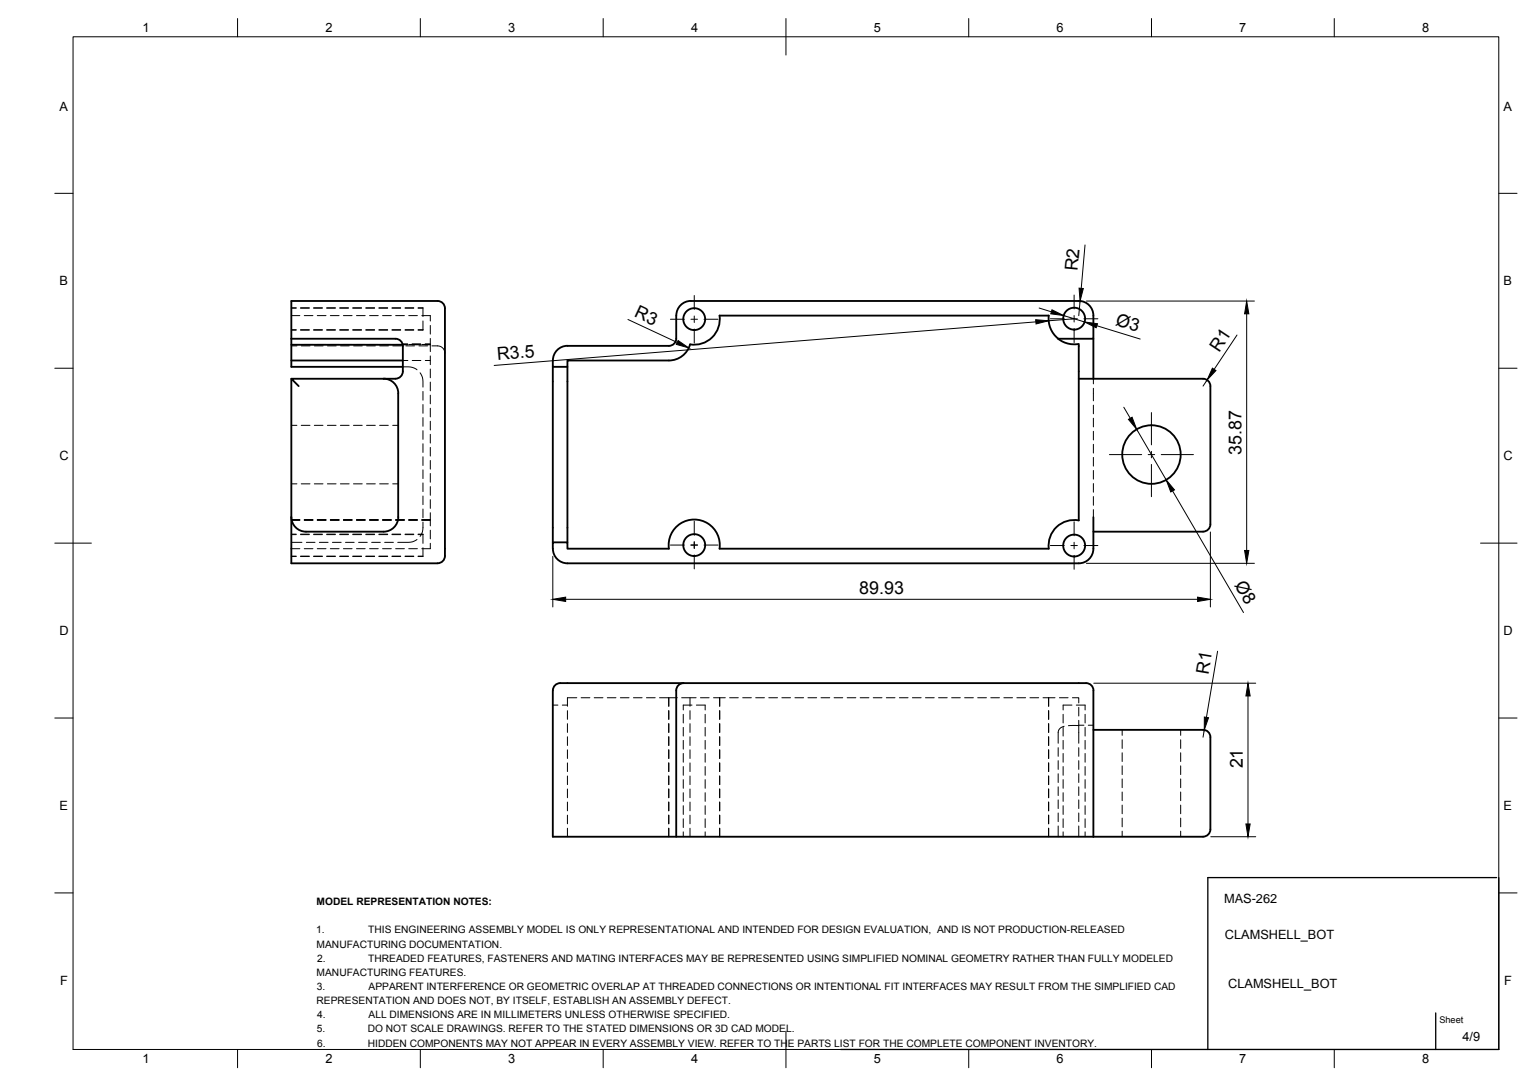
ISO-10303-21;
HEADER;
/* Generated by software containing ST-Developer
 * from STEP Tools, Inc. (www.steptools.com) 
 */

FILE_DESCRIPTION(
/* description */ (''),
/* implementation_level */ '2;1');

FILE_NAME(
/* name */ 'CLAMSHELL_BOT.step',
/* time_stamp */ '2026-10-07T02:13:48+06:00',
/* author */ (''),
/* organization */ (''),
/* preprocessor_version */ 'ST-DEVELOPER v20.2',
/* originating_system */ 'Autodesk Translation Framework v15.15.0.0',
/* authorisation */ '');

FILE_SCHEMA (('AUTOMOTIVE_DESIGN { 1 0 10303 214 3 1 1 }'));
ENDSEC;

DATA;
#10=MECHANICAL_DESIGN_GEOMETRIC_PRESENTATION_REPRESENTATION('',(#115),#17042);
#91=SHAPE_REPRESENTATION_RELATIONSHIP('SRR','None',#17087,#103);
#103=ADVANCED_BREP_SHAPE_REPRESENTATION('',(#127),#17031);
#115=STYLED_ITEM('',(#17154),#127);
#127=MANIFOLD_SOLID_BREP('Body1',#8116);
#142=FACE_BOUND('',#1059,.T.);
#143=FACE_BOUND('',#1060,.T.);
#144=FACE_BOUND('',#1071,.T.);
#145=FACE_BOUND('',#1079,.T.);
#146=FACE_BOUND('',#1085,.T.);
#147=FACE_BOUND('',#1086,.T.);
#180=(
BOUNDED_SURFACE()
B_SPLINE_SURFACE(2,2,((#12432,#12433,#12434),(#12435,#12436,#12437),(#12438,
#12439,#12440)),.UNSPECIFIED.,.F.,.F.,.F.)
B_SPLINE_SURFACE_WITH_KNOTS((3,3),(3,3),(0.,1.5707963267949),(-1.5707963267949,
0.),.UNSPECIFIED.)
GEOMETRIC_REPRESENTATION_ITEM()
RATIONAL_B_SPLINE_SURFACE(((1.,0.707106781186548,1.),(0.707106781186545,
0.499999999999998,0.707106781186545),(1.,0.707106781186548,1.)))
REPRESENTATION_ITEM('')
SURFACE()
);
#181=(
BOUNDED_SURFACE()
B_SPLINE_SURFACE(2,2,((#12455,#12456,#12457),(#12458,#12459,#12460),(#12461,
#12462,#12463)),.UNSPECIFIED.,.F.,.F.,.F.)
B_SPLINE_SURFACE_WITH_KNOTS((3,3),(3,3),(0.,1.5707963267949),(0.,1.5707963267949),
 .UNSPECIFIED.)
GEOMETRIC_REPRESENTATION_ITEM()
RATIONAL_B_SPLINE_SURFACE(((1.,0.707106781186548,1.),(0.707106781186551,
0.500000000000003,0.707106781186551),(1.,0.707106781186548,1.)))
REPRESENTATION_ITEM('')
SURFACE()
);
#182=(
BOUNDED_SURFACE()
B_SPLINE_SURFACE(2,2,((#12484,#12485,#12486),(#12487,#12488,#12489),(#12490,
#12491,#12492)),.UNSPECIFIED.,.F.,.F.,.F.)
B_SPLINE_SURFACE_WITH_KNOTS((3,3),(3,3),(-1.5707963267949,0.),(-1.5707963267949,
0.),.UNSPECIFIED.)
GEOMETRIC_REPRESENTATION_ITEM()
RATIONAL_B_SPLINE_SURFACE(((1.,0.707106781186548,1.),(0.707106781186551,
0.500000000000002,0.707106781186551),(1.,0.707106781186548,1.)))
REPRESENTATION_ITEM('')
SURFACE()
);
#183=(
BOUNDED_SURFACE()
B_SPLINE_SURFACE(2,2,((#12730,#12731,#12732),(#12733,#12734,#12735),(#12736,
#12737,#12738)),.UNSPECIFIED.,.F.,.F.,.F.)
B_SPLINE_SURFACE_WITH_KNOTS((3,3),(3,3),(0.,1.5707963267949),(-4.44089209850066E-15,
1.57079632679491),.UNSPECIFIED.)
GEOMETRIC_REPRESENTATION_ITEM()
RATIONAL_B_SPLINE_SURFACE(((1.,0.707106781186543,1.),(0.707106781186536,
0.499999999999988,0.707106781186536),(1.,0.707106781186543,1.)))
REPRESENTATION_ITEM('')
SURFACE()
);
#184=(
BOUNDED_SURFACE()
B_SPLINE_SURFACE(2,2,((#12750,#12751,#12752),(#12753,#12754,#12755),(#12756,
#12757,#12758)),.UNSPECIFIED.,.F.,.F.,.F.)
B_SPLINE_SURFACE_WITH_KNOTS((3,3),(3,3),(0.,1.5707963267949),(1.57079632679489,
3.14159265358979),.UNSPECIFIED.)
GEOMETRIC_REPRESENTATION_ITEM()
RATIONAL_B_SPLINE_SURFACE(((1.,0.707106781186546,1.),(0.707106781186536,
0.499999999999991,0.707106781186536),(1.,0.707106781186546,1.)))
REPRESENTATION_ITEM('')
SURFACE()
);
#185=(
BOUNDED_SURFACE()
B_SPLINE_SURFACE(2,2,((#12767,#12768,#12769),(#12770,#12771,#12772),(#12773,
#12774,#12775)),.UNSPECIFIED.,.F.,.F.,.F.)
B_SPLINE_SURFACE_WITH_KNOTS((3,3),(3,3),(0.,1.5707963267949),(-3.14159265358979,
-1.5707963267949),.UNSPECIFIED.)
GEOMETRIC_REPRESENTATION_ITEM()
RATIONAL_B_SPLINE_SURFACE(((1.,0.707106781186547,1.),(0.707106781186536,
0.499999999999992,0.707106781186536),(1.,0.707106781186547,1.)))
REPRESENTATION_ITEM('')
SURFACE()
);
#186=(
BOUNDED_SURFACE()
B_SPLINE_SURFACE(2,2,((#12787,#12788,#12789),(#12790,#12791,#12792),(#12793,
#12794,#12795)),.UNSPECIFIED.,.F.,.F.,.F.)
B_SPLINE_SURFACE_WITH_KNOTS((3,3),(3,3),(0.,1.5707963267949),(-1.5707963267949,
-1.11022302462516E-15),.UNSPECIFIED.)
GEOMETRIC_REPRESENTATION_ITEM()
RATIONAL_B_SPLINE_SURFACE(((1.,0.707106781186548,1.),(0.707106781186552,
0.500000000000004,0.707106781186552),(1.,0.707106781186548,1.)))
REPRESENTATION_ITEM('')
SURFACE()
);
#187=(
BOUNDED_SURFACE()
B_SPLINE_SURFACE(2,2,((#12804,#12805,#12806),(#12807,#12808,#12809),(#12810,
#12811,#12812)),.UNSPECIFIED.,.F.,.F.,.F.)
B_SPLINE_SURFACE_WITH_KNOTS((3,3),(3,3),(0.,1.5707963267949),(1.11022302462515E-15,
1.57079632679489),.UNSPECIFIED.)
GEOMETRIC_REPRESENTATION_ITEM()
RATIONAL_B_SPLINE_SURFACE(((1.,0.707106781186549,1.),(0.707106781186552,
0.500000000000005,0.707106781186552),(1.,0.707106781186549,1.)))
REPRESENTATION_ITEM('')
SURFACE()
);
#219=TOROIDAL_SURFACE('',#8562,2.,1.);
#239=ELLIPSE('',#8484,1.4142135623731,1.);
#330=PLANE('',#8463);
#331=PLANE('',#8491);
#332=PLANE('',#8494);
#333=PLANE('',#8496);
#334=PLANE('',#8500);
#335=PLANE('',#8501);
#336=PLANE('',#8506);
#337=PLANE('',#8507);
#338=PLANE('',#8508);
#339=PLANE('',#8513);
#340=PLANE('',#8523);
#341=PLANE('',#8524);
#342=PLANE('',#8528);
#343=PLANE('',#8529);
#344=PLANE('',#8530);
#345=PLANE('',#8531);
#346=PLANE('',#8537);
#347=PLANE('',#8538);
#348=PLANE('',#8539);
#349=PLANE('',#8541);
#350=PLANE('',#8546);
#351=PLANE('',#8549);
#352=PLANE('',#8552);
#353=PLANE('',#8555);
#354=PLANE('',#8558);
#355=PLANE('',#8591);
#356=PLANE('',#8593);
#357=PLANE('',#8595);
#358=PLANE('',#8596);
#359=PLANE('',#8599);
#577=FACE_OUTER_BOUND('',#1058,.T.);
#578=FACE_OUTER_BOUND('',#1061,.T.);
#579=FACE_OUTER_BOUND('',#1062,.T.);
#580=FACE_OUTER_BOUND('',#1063,.T.);
#581=FACE_OUTER_BOUND('',#1064,.T.);
#582=FACE_OUTER_BOUND('',#1065,.T.);
#583=FACE_OUTER_BOUND('',#1066,.T.);
#584=FACE_OUTER_BOUND('',#1067,.T.);
#585=FACE_OUTER_BOUND('',#1068,.T.);
#586=FACE_OUTER_BOUND('',#1069,.T.);
#587=FACE_OUTER_BOUND('',#1070,.T.);
#588=FACE_OUTER_BOUND('',#1072,.T.);
#589=FACE_OUTER_BOUND('',#1073,.T.);
#590=FACE_OUTER_BOUND('',#1074,.T.);
#591=FACE_OUTER_BOUND('',#1075,.T.);
#592=FACE_OUTER_BOUND('',#1076,.T.);
#593=FACE_OUTER_BOUND('',#1077,.T.);
#594=FACE_OUTER_BOUND('',#1078,.T.);
#595=FACE_OUTER_BOUND('',#1080,.T.);
#596=FACE_OUTER_BOUND('',#1081,.T.);
#597=FACE_OUTER_BOUND('',#1082,.T.);
#598=FACE_OUTER_BOUND('',#1083,.T.);
#599=FACE_OUTER_BOUND('',#1084,.T.);
#600=FACE_OUTER_BOUND('',#1087,.T.);
#601=FACE_OUTER_BOUND('',#1088,.T.);
#602=FACE_OUTER_BOUND('',#1089,.T.);
#603=FACE_OUTER_BOUND('',#1090,.T.);
#604=FACE_OUTER_BOUND('',#1091,.T.);
#605=FACE_OUTER_BOUND('',#1092,.T.);
#606=FACE_OUTER_BOUND('',#1093,.T.);
#607=FACE_OUTER_BOUND('',#1094,.T.);
#608=FACE_OUTER_BOUND('',#1095,.T.);
#609=FACE_OUTER_BOUND('',#1096,.T.);
#610=FACE_OUTER_BOUND('',#1097,.T.);
#611=FACE_OUTER_BOUND('',#1098,.T.);
#612=FACE_OUTER_BOUND('',#1099,.T.);
#613=FACE_OUTER_BOUND('',#1100,.T.);
#614=FACE_OUTER_BOUND('',#1101,.T.);
#615=FACE_OUTER_BOUND('',#1102,.T.);
#616=FACE_OUTER_BOUND('',#1103,.T.);
#617=FACE_OUTER_BOUND('',#1104,.T.);
#618=FACE_OUTER_BOUND('',#1105,.T.);
#619=FACE_OUTER_BOUND('',#1106,.T.);
#620=FACE_OUTER_BOUND('',#1107,.T.);
#621=FACE_OUTER_BOUND('',#1108,.T.);
#622=FACE_OUTER_BOUND('',#1109,.T.);
#623=FACE_OUTER_BOUND('',#1110,.T.);
#624=FACE_OUTER_BOUND('',#1111,.T.);
#625=FACE_OUTER_BOUND('',#1112,.T.);
#626=FACE_OUTER_BOUND('',#1113,.T.);
#627=FACE_OUTER_BOUND('',#1114,.T.);
#628=FACE_OUTER_BOUND('',#1115,.T.);
#629=FACE_OUTER_BOUND('',#1116,.T.);
#630=FACE_OUTER_BOUND('',#1117,.T.);
#631=FACE_OUTER_BOUND('',#1118,.T.);
#632=FACE_OUTER_BOUND('',#1119,.T.);
#633=FACE_OUTER_BOUND('',#1120,.T.);
#634=FACE_OUTER_BOUND('',#1121,.T.);
#635=FACE_OUTER_BOUND('',#1122,.T.);
#636=FACE_OUTER_BOUND('',#1123,.T.);
#637=FACE_OUTER_BOUND('',#1124,.T.);
#638=FACE_OUTER_BOUND('',#1125,.T.);
#639=FACE_OUTER_BOUND('',#1126,.T.);
#640=FACE_OUTER_BOUND('',#1127,.T.);
#641=FACE_OUTER_BOUND('',#1128,.T.);
#642=FACE_OUTER_BOUND('',#1129,.T.);
#643=FACE_OUTER_BOUND('',#1130,.T.);
#644=FACE_OUTER_BOUND('',#1131,.T.);
#645=FACE_OUTER_BOUND('',#1132,.T.);
#646=FACE_OUTER_BOUND('',#1133,.T.);
#647=FACE_OUTER_BOUND('',#1134,.T.);
#648=FACE_OUTER_BOUND('',#1135,.T.);
#1058=EDGE_LOOP('',(#5643,#5644,#5645,#5646,#5647,#5648,#5649,#5650,#5651,
#5652,#5653,#5654,#5655,#5656,#5657,#5658,#5659));
#1059=EDGE_LOOP('',(#5660));
#1060=EDGE_LOOP('',(#5661));
#1061=EDGE_LOOP('',(#5662,#5663,#5664,#5665));
#1062=EDGE_LOOP('',(#5666,#5667,#5668,#5669));
#1063=EDGE_LOOP('',(#5670,#5671,#5672,#5673));
#1064=EDGE_LOOP('',(#5674,#5675,#5676,#5677));
#1065=EDGE_LOOP('',(#5678,#5679,#5680,#5681));
#1066=EDGE_LOOP('',(#5682,#5683,#5684,#5685));
#1067=EDGE_LOOP('',(#5686,#5687,#5688,#5689));
#1068=EDGE_LOOP('',(#5690,#5691,#5692,#5693));
#1069=EDGE_LOOP('',(#5694,#5695,#5696,#5697,#5698));
#1070=EDGE_LOOP('',(#5699,#5700,#5701,#5702));
#1071=EDGE_LOOP('',(#5703));
#1072=EDGE_LOOP('',(#5704,#5705,#5706,#5707,#5708,#5709,#5710));
#1073=EDGE_LOOP('',(#5711,#5712,#5713,#5714));
#1074=EDGE_LOOP('',(#5715,#5716,#5717,#5718));
#1075=EDGE_LOOP('',(#5719,#5720,#5721,#5722,#5723,#5724,#5725));
#1076=EDGE_LOOP('',(#5726,#5727,#5728,#5729,#5730,#5731,#5732,#5733,#5734,
#5735,#5736,#5737,#5738,#5739,#5740));
#1077=EDGE_LOOP('',(#5741,#5742,#5743,#5744));
#1078=EDGE_LOOP('',(#5745,#5746,#5747,#5748));
#1079=EDGE_LOOP('',(#5749));
#1080=EDGE_LOOP('',(#5750,#5751,#5752,#5753));
#1081=EDGE_LOOP('',(#5754,#5755,#5756,#5757));
#1082=EDGE_LOOP('',(#5758,#5759,#5760,#5761,#5762));
#1083=EDGE_LOOP('',(#5763,#5764,#5765,#5766));
#1084=EDGE_LOOP('',(#5767,#5768,#5769,#5770,#5771,#5772,#5773,#5774,#5775,
#5776,#5777,#5778,#5779,#5780,#5781));
#1085=EDGE_LOOP('',(#5782));
#1086=EDGE_LOOP('',(#5783));
#1087=EDGE_LOOP('',(#5784,#5785,#5786,#5787));
#1088=EDGE_LOOP('',(#5788,#5789,#5790,#5791));
#1089=EDGE_LOOP('',(#5792,#5793,#5794,#5795));
#1090=EDGE_LOOP('',(#5796,#5797,#5798,#5799));
#1091=EDGE_LOOP('',(#5800,#5801,#5802,#5803));
#1092=EDGE_LOOP('',(#5804,#5805,#5806,#5807,#5808,#5809,#5810,#5811,#5812,
#5813));
#1093=EDGE_LOOP('',(#5814,#5815,#5816,#5817,#5818,#5819,#5820,#5821));
#1094=EDGE_LOOP('',(#5822,#5823,#5824,#5825,#5826,#5827,#5828,#5829,#5830,
#5831,#5832));
#1095=EDGE_LOOP('',(#5833,#5834,#5835,#5836));
#1096=EDGE_LOOP('',(#5837,#5838,#5839,#5840));
#1097=EDGE_LOOP('',(#5841,#5842,#5843,#5844));
#1098=EDGE_LOOP('',(#5845,#5846,#5847,#5848));
#1099=EDGE_LOOP('',(#5849,#5850,#5851,#5852,#5853,#5854,#5855,#5856,#5857,
#5858));
#1100=EDGE_LOOP('',(#5859,#5860,#5861,#5862));
#1101=EDGE_LOOP('',(#5863,#5864,#5865,#5866));
#1102=EDGE_LOOP('',(#5867,#5868,#5869,#5870));
#1103=EDGE_LOOP('',(#5871,#5872,#5873,#5874,#5875,#5876));
#1104=EDGE_LOOP('',(#5877,#5878,#5879,#5880));
#1105=EDGE_LOOP('',(#5881,#5882,#5883,#5884));
#1106=EDGE_LOOP('',(#5885));
#1107=EDGE_LOOP('',(#5886,#5887,#5888,#5889));
#1108=EDGE_LOOP('',(#5890));
#1109=EDGE_LOOP('',(#5891,#5892,#5893,#5894));
#1110=EDGE_LOOP('',(#5895));
#1111=EDGE_LOOP('',(#5896,#5897,#5898,#5899));
#1112=EDGE_LOOP('',(#5900));
#1113=EDGE_LOOP('',(#5901,#5902,#5903,#5904));
#1114=EDGE_LOOP('',(#5905,#5906,#5907,#5908));
#1115=EDGE_LOOP('',(#5909,#5910,#5911,#5912));
#1116=EDGE_LOOP('',(#5913,#5914,#5915,#5916));
#1117=EDGE_LOOP('',(#5917,#5918,#5919,#5920));
#1118=EDGE_LOOP('',(#5921,#5922,#5923,#5924));
#1119=EDGE_LOOP('',(#5925,#5926,#5927,#5928));
#1120=EDGE_LOOP('',(#5929,#5930,#5931,#5932));
#1121=EDGE_LOOP('',(#5933,#5934,#5935,#5936));
#1122=EDGE_LOOP('',(#5937,#5938,#5939,#5940));
#1123=EDGE_LOOP('',(#5941,#5942,#5943,#5944));
#1124=EDGE_LOOP('',(#5945,#5946,#5947,#5948));
#1125=EDGE_LOOP('',(#5949,#5950,#5951,#5952));
#1126=EDGE_LOOP('',(#5953,#5954,#5955,#5956));
#1127=EDGE_LOOP('',(#5957,#5958,#5959,#5960));
#1128=EDGE_LOOP('',(#5961,#5962,#5963,#5964));
#1129=EDGE_LOOP('',(#5965,#5966,#5967,#5968));
#1130=EDGE_LOOP('',(#5969,#5970,#5971,#5972));
#1131=EDGE_LOOP('',(#5973,#5974,#5975,#5976,#5977,#5978,#5979,#5980,#5981,
#5982,#5983,#5984));
#1132=EDGE_LOOP('',(#5985,#5986,#5987,#5988));
#1133=EDGE_LOOP('',(#5989,#5990,#5991,#5992));
#1134=EDGE_LOOP('',(#5993,#5994,#5995,#5996));
#1135=EDGE_LOOP('',(#5997,#5998,#5999,#6000));
#1569=CIRCLE('',#8464,2.);
#1570=CIRCLE('',#8465,1.99999999999999);
#1571=CIRCLE('',#8466,0.999999999999996);
#1572=CIRCLE('',#8467,2.00000000000001);
#1573=CIRCLE('',#8468,3.);
#1574=CIRCLE('',#8469,3.5);
#1575=CIRCLE('',#8470,3.5);
#1576=CIRCLE('',#8471,1.5);
#1577=CIRCLE('',#8472,1.5);
#1578=CIRCLE('',#8473,1.);
#1579=CIRCLE('',#8474,2.);
#1580=CIRCLE('',#8475,1.);
#1581=CIRCLE('',#8476,1.);
#1582=CIRCLE('',#8478,1.);
#1583=CIRCLE('',#8479,1.);
#1584=CIRCLE('',#8480,2.);
#1585=CIRCLE('',#8481,1.);
#1586=CIRCLE('',#8482,1.);
#1587=CIRCLE('',#8486,1.);
#1588=CIRCLE('',#8487,2.);
#1589=CIRCLE('',#8488,1.);
#1590=CIRCLE('',#8490,2.);
#1591=CIRCLE('',#8493,2.);
#1592=CIRCLE('',#8495,4.);
#1593=CIRCLE('',#8499,2.);
#1594=CIRCLE('',#8502,0.999999999999999);
#1595=CIRCLE('',#8503,1.);
#1596=CIRCLE('',#8505,4.);
#1597=CIRCLE('',#8510,0.999999999999999);
#1598=CIRCLE('',#8512,1.);
#1599=CIRCLE('',#8514,3.5);
#1600=CIRCLE('',#8515,3.5);
#1601=CIRCLE('',#8516,2.);
#1602=CIRCLE('',#8517,2.);
#1603=CIRCLE('',#8518,1.5);
#1604=CIRCLE('',#8519,1.5);
#1605=CIRCLE('',#8521,2.);
#1606=CIRCLE('',#8522,2.);
#1607=CIRCLE('',#8526,2.);
#1608=CIRCLE('',#8527,2.);
#1609=CIRCLE('',#8532,3.5);
#1610=CIRCLE('',#8533,3.5);
#1611=CIRCLE('',#8534,3.);
#1612=CIRCLE('',#8535,3.5);
#1613=CIRCLE('',#8536,3.5);
#1614=CIRCLE('',#8548,1.5);
#1615=CIRCLE('',#8551,1.5);
#1616=CIRCLE('',#8554,1.5);
#1617=CIRCLE('',#8557,1.5);
#1618=CIRCLE('',#8560,1.);
#1619=CIRCLE('',#8561,1.);
#1620=CIRCLE('',#8563,0.999999999999996);
#1621=CIRCLE('',#8564,2.);
#1622=CIRCLE('',#8565,0.999999999999996);
#1623=CIRCLE('',#8567,0.999999999999996);
#1624=CIRCLE('',#8568,1.);
#1625=CIRCLE('',#8569,0.999999999999993);
#1626=CIRCLE('',#8570,1.99999999999999);
#1627=CIRCLE('',#8572,1.);
#1628=CIRCLE('',#8573,1.);
#1629=CIRCLE('',#8574,0.999999999999997);
#1630=CIRCLE('',#8575,2.);
#1631=CIRCLE('',#8577,1.);
#1632=CIRCLE('',#8578,0.999999999999999);
#1633=CIRCLE('',#8579,0.999999999999998);
#1634=CIRCLE('',#8580,2.);
#1635=CIRCLE('',#8582,0.999999999999999);
#1636=CIRCLE('',#8583,0.999999999999996);
#1637=CIRCLE('',#8584,1.);
#1638=CIRCLE('',#8585,2.);
#1639=CIRCLE('',#8587,0.999999999999996);
#1640=CIRCLE('',#8588,1.00000000000001);
#1641=CIRCLE('',#8589,2.00000000000001);
#1951=B_SPLINE_CURVE_WITH_KNOTS('',3,(#12568,#12569,#12570,#12571,#12572,
#12573,#12574,#12575,#12576,#12577,#12578,#12579,#12580,#12581),
 .UNSPECIFIED.,.F.,.F.,(4,2,2,2,2,2,4),(0.243709125451541,0.275010306594212,
0.329604611857381,0.356901764488965,0.38419891712055,0.398357188505934,
0.412515459891318),.UNSPECIFIED.);
#2197=LINE('',#12396,#2775);
#2198=LINE('',#12398,#2776);
#2199=LINE('',#12402,#2777);
#2200=LINE('',#12406,#2778);
#2201=LINE('',#12410,#2779);
#2202=LINE('',#12414,#2780);
#2203=LINE('',#12416,#2781);
#2204=LINE('',#12418,#2782);
#2205=LINE('',#12420,#2783);
#2206=LINE('',#12426,#2784);
#2207=LINE('',#12453,#2785);
#2208=LINE('',#12454,#2786);
#2209=LINE('',#12474,#2787);
#2210=LINE('',#12476,#2788);
#2211=LINE('',#12480,#2789);
#2212=LINE('',#12483,#2790);
#2213=LINE('',#12497,#2791);
#2214=LINE('',#12500,#2792);
#2215=LINE('',#12503,#2793);
#2216=LINE('',#12504,#2794);
#2217=LINE('',#12507,#2795);
#2218=LINE('',#12509,#2796);
#2219=LINE('',#12513,#2797);
#2220=LINE('',#12514,#2798);
#2221=LINE('',#12519,#2799);
#2222=LINE('',#12521,#2800);
#2223=LINE('',#12523,#2801);
#2224=LINE('',#12525,#2802);
#2225=LINE('',#12526,#2803);
#2226=LINE('',#12528,#2804);
#2227=LINE('',#12529,#2805);
#2228=LINE('',#12532,#2806);
#2229=LINE('',#12537,#2807);
#2230=LINE('',#12539,#2808);
#2231=LINE('',#12541,#2809);
#2232=LINE('',#12542,#2810);
#2233=LINE('',#12544,#2811);
#2234=LINE('',#12548,#2812);
#2235=LINE('',#12550,#2813);
#2236=LINE('',#12554,#2814);
#2237=LINE('',#12558,#2815);
#2238=LINE('',#12559,#2816);
#2239=LINE('',#12562,#2817);
#2240=LINE('',#12564,#2818);
#2241=LINE('',#12565,#2819);
#2242=LINE('',#12587,#2820);
#2243=LINE('',#12591,#2821);
#2244=LINE('',#12595,#2822);
#2245=LINE('',#12597,#2823);
#2246=LINE('',#12599,#2824);
#2247=LINE('',#12601,#2825);
#2248=LINE('',#12605,#2826);
#2249=LINE('',#12616,#2827);
#2250=LINE('',#12619,#2828);
#2251=LINE('',#12621,#2829);
#2252=LINE('',#12622,#2830);
#2253=LINE('',#12625,#2831);
#2254=LINE('',#12627,#2832);
#2255=LINE('',#12628,#2833);
#2256=LINE('',#12634,#2834);
#2257=LINE('',#12636,#2835);
#2258=LINE('',#12637,#2836);
#2259=LINE('',#12640,#2837);
#2260=LINE('',#12642,#2838);
#2261=LINE('',#12643,#2839);
#2262=LINE('',#12646,#2840);
#2263=LINE('',#12648,#2841);
#2264=LINE('',#12649,#2842);
#2265=LINE('',#12654,#2843);
#2266=LINE('',#12660,#2844);
#2267=LINE('',#12662,#2845);
#2268=LINE('',#12664,#2846);
#2269=LINE('',#12668,#2847);
#2270=LINE('',#12671,#2848);
#2271=LINE('',#12672,#2849);
#2272=LINE('',#12674,#2850);
#2273=LINE('',#12675,#2851);
#2274=LINE('',#12677,#2852);
#2275=LINE('',#12678,#2853);
#2276=LINE('',#12680,#2854);
#2277=LINE('',#12681,#2855);
#2278=LINE('',#12683,#2856);
#2279=LINE('',#12691,#2857);
#2280=LINE('',#12696,#2858);
#2281=LINE('',#12701,#2859);
#2282=LINE('',#12706,#2860);
#2283=LINE('',#12714,#2861);
#2284=LINE('',#12717,#2862);
#2285=LINE('',#12728,#2863);
#2286=LINE('',#12729,#2864);
#2287=LINE('',#12748,#2865);
#2288=LINE('',#12749,#2866);
#2289=LINE('',#12766,#2867);
#2290=LINE('',#12785,#2868);
#2291=LINE('',#12786,#2869);
#2292=LINE('',#12803,#2870);
#2293=LINE('',#12816,#2871);
#2294=LINE('',#12818,#2872);
#2295=LINE('',#12820,#2873);
#2296=LINE('',#12822,#2874);
#2297=LINE('',#12824,#2875);
#2298=LINE('',#12826,#2876);
#2299=LINE('',#12830,#2877);
#2300=LINE('',#12832,#2878);
#2775=VECTOR('',#9834,20.);
#2776=VECTOR('',#9835,20.);
#2777=VECTOR('',#9838,20.);
#2778=VECTOR('',#9841,20.);
#2779=VECTOR('',#9844,20.);
#2780=VECTOR('',#9847,20.);
#2781=VECTOR('',#9848,20.);
#2782=VECTOR('',#9849,20.);
#2783=VECTOR('',#9850,20.);
#2784=VECTOR('',#9855,20.);
#2785=VECTOR('',#9874,20.);
#2786=VECTOR('',#9875,20.);
#2787=VECTOR('',#9886,20.);
#2788=VECTOR('',#9887,20.);
#2789=VECTOR('',#9892,20.);
#2790=VECTOR('',#9895,20.);
#2791=VECTOR('',#9902,20.);
#2792=VECTOR('',#9905,20.);
#2793=VECTOR('',#9908,20.);
#2794=VECTOR('',#9909,20.);
#2795=VECTOR('',#9912,20.);
#2796=VECTOR('',#9913,20.);
#2797=VECTOR('',#9918,20.);
#2798=VECTOR('',#9919,20.);
#2799=VECTOR('',#9924,20.);
#2800=VECTOR('',#9925,20.);
#2801=VECTOR('',#9926,20.);
#2802=VECTOR('',#9927,20.);
#2803=VECTOR('',#9928,20.);
#2804=VECTOR('',#9931,20.);
#2805=VECTOR('',#9932,20.);
#2806=VECTOR('',#9935,20.);
#2807=VECTOR('',#9942,20.);
#2808=VECTOR('',#9943,20.);
#2809=VECTOR('',#9944,20.);
#2810=VECTOR('',#9945,20.);
#2811=VECTOR('',#9946,20.);
#2812=VECTOR('',#9949,20.);
#2813=VECTOR('',#9952,20.);
#2814=VECTOR('',#9957,4.);
#2815=VECTOR('',#9962,20.);
#2816=VECTOR('',#9963,20.);
#2817=VECTOR('',#9966,20.);
#2818=VECTOR('',#9967,20.);
#2819=VECTOR('',#9968,20.);
#2820=VECTOR('',#9979,20.);
#2821=VECTOR('',#9982,20.);
#2822=VECTOR('',#9985,20.);
#2823=VECTOR('',#9986,20.);
#2824=VECTOR('',#9987,20.);
#2825=VECTOR('',#9988,20.);
#2826=VECTOR('',#9991,20.);
#2827=VECTOR('',#10002,20.);
#2828=VECTOR('',#10005,20.);
#2829=VECTOR('',#10008,20.);
#2830=VECTOR('',#10009,20.);
#2831=VECTOR('',#10012,20.);
#2832=VECTOR('',#10013,20.);
#2833=VECTOR('',#10014,20.);
#2834=VECTOR('',#10021,20.);
#2835=VECTOR('',#10024,20.);
#2836=VECTOR('',#10025,20.);
#2837=VECTOR('',#10028,20.);
#2838=VECTOR('',#10029,20.);
#2839=VECTOR('',#10030,20.);
#2840=VECTOR('',#10033,20.);
#2841=VECTOR('',#10034,20.);
#2842=VECTOR('',#10035,20.);
#2843=VECTOR('',#10040,20.);
#2844=VECTOR('',#10045,20.);
#2845=VECTOR('',#10046,20.);
#2846=VECTOR('',#10047,20.);
#2847=VECTOR('',#10050,20.);
#2848=VECTOR('',#10055,20.);
#2849=VECTOR('',#10056,20.);
#2850=VECTOR('',#10059,20.);
#2851=VECTOR('',#10060,20.);
#2852=VECTOR('',#10063,20.);
#2853=VECTOR('',#10064,20.);
#2854=VECTOR('',#10067,20.);
#2855=VECTOR('',#10068,20.);
#2856=VECTOR('',#10071,20.);
#2857=VECTOR('',#10084,1.5);
#2858=VECTOR('',#10091,1.5);
#2859=VECTOR('',#10098,1.5);
#2860=VECTOR('',#10105,1.5);
#2861=VECTOR('',#10114,20.);
#2862=VECTOR('',#10117,20.);
#2863=VECTOR('',#10130,20.);
#2864=VECTOR('',#10131,20.);
#2865=VECTOR('',#10142,20.);
#2866=VECTOR('',#10143,20.);
#2867=VECTOR('',#10154,20.);
#2868=VECTOR('',#10165,20.);
#2869=VECTOR('',#10166,20.);
#2870=VECTOR('',#10177,20.);
#2871=VECTOR('',#10184,20.);
#2872=VECTOR('',#10187,20.);
#2873=VECTOR('',#10190,20.);
#2874=VECTOR('',#10193,20.);
#2875=VECTOR('',#10196,20.);
#2876=VECTOR('',#10199,20.);
#2877=VECTOR('',#10206,20.);
#2878=VECTOR('',#10209,20.);
#3352=VERTEX_POINT('',#12394);
#3353=VERTEX_POINT('',#12395);
#3354=VERTEX_POINT('',#12397);
#3355=VERTEX_POINT('',#12399);
#3356=VERTEX_POINT('',#12401);
#3357=VERTEX_POINT('',#12403);
#3358=VERTEX_POINT('',#12405);
#3359=VERTEX_POINT('',#12407);
#3360=VERTEX_POINT('',#12409);
#3361=VERTEX_POINT('',#12411);
#3362=VERTEX_POINT('',#12413);
#3363=VERTEX_POINT('',#12415);
#3364=VERTEX_POINT('',#12417);
#3365=VERTEX_POINT('',#12419);
#3366=VERTEX_POINT('',#12421);
#3367=VERTEX_POINT('',#12423);
#3368=VERTEX_POINT('',#12425);
#3369=VERTEX_POINT('',#12428);
#3370=VERTEX_POINT('',#12430);
#3371=VERTEX_POINT('',#12441);
#3372=VERTEX_POINT('',#12442);
#3373=VERTEX_POINT('',#12444);
#3374=VERTEX_POINT('',#12446);
#3375=VERTEX_POINT('',#12450);
#3376=VERTEX_POINT('',#12451);
#3377=VERTEX_POINT('',#12464);
#3378=VERTEX_POINT('',#12465);
#3379=VERTEX_POINT('',#12467);
#3380=VERTEX_POINT('',#12469);
#3381=VERTEX_POINT('',#12473);
#3382=VERTEX_POINT('',#12475);
#3383=VERTEX_POINT('',#12479);
#3384=VERTEX_POINT('',#12481);
#3385=VERTEX_POINT('',#12496);
#3386=VERTEX_POINT('',#12498);
#3387=VERTEX_POINT('',#12502);
#3388=VERTEX_POINT('',#12506);
#3389=VERTEX_POINT('',#12508);
#3390=VERTEX_POINT('',#12512);
#3391=VERTEX_POINT('',#12515);
#3392=VERTEX_POINT('',#12518);
#3393=VERTEX_POINT('',#12520);
#3394=VERTEX_POINT('',#12522);
#3395=VERTEX_POINT('',#12524);
#3396=VERTEX_POINT('',#12531);
#3397=VERTEX_POINT('',#12536);
#3398=VERTEX_POINT('',#12538);
#3399=VERTEX_POINT('',#12540);
#3400=VERTEX_POINT('',#12543);
#3401=VERTEX_POINT('',#12545);
#3402=VERTEX_POINT('',#12547);
#3403=VERTEX_POINT('',#12552);
#3404=VERTEX_POINT('',#12557);
#3405=VERTEX_POINT('',#12561);
#3406=VERTEX_POINT('',#12563);
#3407=VERTEX_POINT('',#12567);
#3408=VERTEX_POINT('',#12586);
#3409=VERTEX_POINT('',#12588);
#3410=VERTEX_POINT('',#12590);
#3411=VERTEX_POINT('',#12592);
#3412=VERTEX_POINT('',#12594);
#3413=VERTEX_POINT('',#12596);
#3414=VERTEX_POINT('',#12598);
#3415=VERTEX_POINT('',#12600);
#3416=VERTEX_POINT('',#12602);
#3417=VERTEX_POINT('',#12604);
#3418=VERTEX_POINT('',#12607);
#3419=VERTEX_POINT('',#12609);
#3420=VERTEX_POINT('',#12612);
#3421=VERTEX_POINT('',#12613);
#3422=VERTEX_POINT('',#12615);
#3423=VERTEX_POINT('',#12617);
#3424=VERTEX_POINT('',#12624);
#3425=VERTEX_POINT('',#12626);
#3426=VERTEX_POINT('',#12630);
#3427=VERTEX_POINT('',#12632);
#3428=VERTEX_POINT('',#12639);
#3429=VERTEX_POINT('',#12641);
#3430=VERTEX_POINT('',#12645);
#3431=VERTEX_POINT('',#12647);
#3432=VERTEX_POINT('',#12651);
#3433=VERTEX_POINT('',#12653);
#3434=VERTEX_POINT('',#12655);
#3435=VERTEX_POINT('',#12657);
#3436=VERTEX_POINT('',#12659);
#3437=VERTEX_POINT('',#12661);
#3438=VERTEX_POINT('',#12663);
#3439=VERTEX_POINT('',#12665);
#3440=VERTEX_POINT('',#12667);
#3441=VERTEX_POINT('',#12690);
#3442=VERTEX_POINT('',#12695);
#3443=VERTEX_POINT('',#12700);
#3444=VERTEX_POINT('',#12705);
#3445=VERTEX_POINT('',#12710);
#3446=VERTEX_POINT('',#12711);
#3447=VERTEX_POINT('',#12713);
#3448=VERTEX_POINT('',#12715);
#3449=VERTEX_POINT('',#12719);
#3450=VERTEX_POINT('',#12720);
#3451=VERTEX_POINT('',#12725);
#3452=VERTEX_POINT('',#12726);
#3453=VERTEX_POINT('',#12739);
#3454=VERTEX_POINT('',#12740);
#3455=VERTEX_POINT('',#12745);
#3456=VERTEX_POINT('',#12746);
#3457=VERTEX_POINT('',#12759);
#3458=VERTEX_POINT('',#12764);
#3459=VERTEX_POINT('',#12776);
#3460=VERTEX_POINT('',#12777);
#3461=VERTEX_POINT('',#12782);
#3462=VERTEX_POINT('',#12783);
#3463=VERTEX_POINT('',#12796);
#3464=VERTEX_POINT('',#12801);
#4189=EDGE_CURVE('',#3352,#3353,#2197,.T.);
#4190=EDGE_CURVE('',#3354,#3353,#2198,.T.);
#4191=EDGE_CURVE('',#3355,#3354,#1569,.T.);
#4192=EDGE_CURVE('',#3356,#3355,#2199,.T.);
#4193=EDGE_CURVE('',#3357,#3356,#1570,.T.);
#4194=EDGE_CURVE('',#3358,#3357,#2200,.T.);
#4195=EDGE_CURVE('',#3358,#3359,#1571,.T.);
#4196=EDGE_CURVE('',#3360,#3359,#2201,.T.);
#4197=EDGE_CURVE('',#3361,#3360,#1572,.T.);
#4198=EDGE_CURVE('',#3362,#3361,#2202,.T.);
#4199=EDGE_CURVE('',#3362,#3363,#2203,.T.);
#4200=EDGE_CURVE('',#3363,#3364,#2204,.T.);
#4201=EDGE_CURVE('',#3364,#3365,#2205,.T.);
#4202=EDGE_CURVE('',#3365,#3366,#1573,.T.);
#4203=EDGE_CURVE('',#3366,#3367,#1574,.T.);
#4204=EDGE_CURVE('',#3367,#3368,#2206,.T.);
#4205=EDGE_CURVE('',#3368,#3352,#1575,.T.);
#4206=EDGE_CURVE('',#3369,#3369,#1576,.T.);
#4207=EDGE_CURVE('',#3370,#3370,#1577,.T.);
#4208=EDGE_CURVE('',#3371,#3372,#1578,.T.);
#4209=EDGE_CURVE('',#3372,#3373,#1579,.T.);
#4210=EDGE_CURVE('',#3373,#3374,#1580,.T.);
#4211=EDGE_CURVE('',#3374,#3371,#1581,.T.);
#4212=EDGE_CURVE('',#3375,#3376,#1582,.T.);
#4213=EDGE_CURVE('',#3376,#3372,#2207,.T.);
#4214=EDGE_CURVE('',#3371,#3375,#2208,.T.);
#4215=EDGE_CURVE('',#3377,#3378,#1583,.T.);
#4216=EDGE_CURVE('',#3378,#3379,#1584,.T.);
#4217=EDGE_CURVE('',#3379,#3380,#1585,.T.);
#4218=EDGE_CURVE('',#3380,#3377,#1586,.T.);
#4219=EDGE_CURVE('',#3381,#3380,#2209,.T.);
#4220=EDGE_CURVE('',#3379,#3382,#2210,.T.);
#4221=EDGE_CURVE('',#3382,#3381,#239,.T.);
#4222=EDGE_CURVE('',#3382,#3383,#2211,.T.);
#4223=EDGE_CURVE('',#3383,#3384,#1587,.T.);
#4224=EDGE_CURVE('',#3384,#3381,#2212,.T.);
#4225=EDGE_CURVE('',#3383,#3376,#1588,.T.);
#4226=EDGE_CURVE('',#3375,#3384,#1589,.T.);
#4227=EDGE_CURVE('',#3385,#3372,#2213,.T.);
#4228=EDGE_CURVE('',#3386,#3385,#1590,.T.);
#4229=EDGE_CURVE('',#3386,#3373,#2214,.T.);
#4230=EDGE_CURVE('',#3387,#3376,#2215,.T.);
#4231=EDGE_CURVE('',#3385,#3387,#2216,.T.);
#4232=EDGE_CURVE('',#3383,#3388,#2217,.T.);
#4233=EDGE_CURVE('',#3388,#3389,#2218,.T.);
#4234=EDGE_CURVE('',#3389,#3387,#1591,.F.);
#4235=EDGE_CURVE('',#3390,#3382,#2219,.T.);
#4236=EDGE_CURVE('',#3390,#3388,#2220,.T.);
#4237=EDGE_CURVE('',#3391,#3391,#1592,.F.);
#4238=EDGE_CURVE('',#3392,#3379,#2221,.T.);
#4239=EDGE_CURVE('',#3393,#3392,#2222,.T.);
#4240=EDGE_CURVE('',#3393,#3394,#2223,.T.);
#4241=EDGE_CURVE('',#3395,#3394,#2224,.T.);
#4242=EDGE_CURVE('',#3390,#3395,#2225,.T.);
#4243=EDGE_CURVE('',#3373,#3378,#2226,.T.);
#4244=EDGE_CURVE('',#3377,#3374,#2227,.T.);
#4245=EDGE_CURVE('',#3396,#3378,#2228,.T.);
#4246=EDGE_CURVE('',#3392,#3396,#1593,.T.);
#4247=EDGE_CURVE('',#3389,#3397,#2229,.T.);
#4248=EDGE_CURVE('',#3397,#3398,#2230,.T.);
#4249=EDGE_CURVE('',#3399,#3398,#2231,.T.);
#4250=EDGE_CURVE('',#3354,#3399,#2232,.T.);
#4251=EDGE_CURVE('',#3353,#3400,#2233,.T.);
#4252=EDGE_CURVE('',#3400,#3401,#1594,.T.);
#4253=EDGE_CURVE('',#3401,#3402,#2234,.T.);
#4254=EDGE_CURVE('',#3402,#3393,#1595,.T.);
#4255=EDGE_CURVE('',#3396,#3386,#2235,.T.);
#4256=EDGE_CURVE('',#3403,#3403,#1596,.T.);
#4257=EDGE_CURVE('',#3403,#3391,#2236,.T.);
#4258=EDGE_CURVE('',#3404,#3352,#2237,.T.);
#4259=EDGE_CURVE('',#3400,#3404,#2238,.T.);
#4260=EDGE_CURVE('',#3401,#3405,#2239,.T.);
#4261=EDGE_CURVE('',#3406,#3405,#2240,.T.);
#4262=EDGE_CURVE('',#3402,#3406,#2241,.T.);
#4263=EDGE_CURVE('',#3407,#3404,#1951,.T.);
#4264=EDGE_CURVE('',#3405,#3407,#1597,.T.);
#4265=EDGE_CURVE('',#3394,#3406,#1598,.T.);
#4266=EDGE_CURVE('',#3395,#3408,#2242,.T.);
#4267=EDGE_CURVE('',#3408,#3409,#1599,.T.);
#4268=EDGE_CURVE('',#3409,#3410,#2243,.T.);
#4269=EDGE_CURVE('',#3410,#3411,#1600,.T.);
#4270=EDGE_CURVE('',#3411,#3412,#2244,.T.);
#4271=EDGE_CURVE('',#3412,#3413,#2245,.T.);
#4272=EDGE_CURVE('',#3413,#3414,#2246,.T.);
#4273=EDGE_CURVE('',#3415,#3414,#2247,.T.);
#4274=EDGE_CURVE('',#3416,#3415,#1601,.T.);
#4275=EDGE_CURVE('',#3417,#3416,#2248,.T.);
#4276=EDGE_CURVE('',#3397,#3417,#1602,.T.);
#4277=EDGE_CURVE('',#3418,#3418,#1603,.T.);
#4278=EDGE_CURVE('',#3419,#3419,#1604,.T.);
#4279=EDGE_CURVE('',#3420,#3421,#1605,.T.);
#4280=EDGE_CURVE('',#3422,#3420,#2249,.T.);
#4281=EDGE_CURVE('',#3423,#3422,#1606,.T.);
#4282=EDGE_CURVE('',#3423,#3421,#2250,.T.);
#4283=EDGE_CURVE('',#3421,#3413,#2251,.T.);
#4284=EDGE_CURVE('',#3414,#3423,#2252,.T.);
#4285=EDGE_CURVE('',#3363,#3424,#2253,.T.);
#4286=EDGE_CURVE('',#3425,#3362,#2254,.T.);
#4287=EDGE_CURVE('',#3425,#3424,#2255,.T.);
#4288=EDGE_CURVE('',#3424,#3426,#1607,.T.);
#4289=EDGE_CURVE('',#3427,#3425,#1608,.T.);
#4290=EDGE_CURVE('',#3427,#3426,#2256,.T.);
#4291=EDGE_CURVE('',#3426,#3420,#2257,.T.);
#4292=EDGE_CURVE('',#3422,#3427,#2258,.T.);
#4293=EDGE_CURVE('',#3361,#3428,#2259,.T.);
#4294=EDGE_CURVE('',#3429,#3428,#2260,.T.);
#4295=EDGE_CURVE('',#3415,#3429,#2261,.T.);
#4296=EDGE_CURVE('',#3407,#3430,#2262,.T.);
#4297=EDGE_CURVE('',#3430,#3431,#2263,.T.);
#4298=EDGE_CURVE('',#3431,#3408,#2264,.T.);
#4299=EDGE_CURVE('',#3430,#3432,#1609,.T.);
#4300=EDGE_CURVE('',#3433,#3432,#2265,.F.);
#4301=EDGE_CURVE('',#3433,#3434,#1610,.T.);
#4302=EDGE_CURVE('',#3435,#3434,#1611,.F.);
#4303=EDGE_CURVE('',#3435,#3436,#2266,.T.);
#4304=EDGE_CURVE('',#3437,#3436,#2267,.T.);
#4305=EDGE_CURVE('',#3438,#3437,#2268,.T.);
#4306=EDGE_CURVE('',#3438,#3439,#1612,.T.);
#4307=EDGE_CURVE('',#3440,#3439,#2269,.T.);
#4308=EDGE_CURVE('',#3440,#3431,#1613,.T.);
#4309=EDGE_CURVE('',#3432,#3368,#2270,.T.);
#4310=EDGE_CURVE('',#3367,#3433,#2271,.T.);
#4311=EDGE_CURVE('',#3411,#3438,#2272,.T.);
#4312=EDGE_CURVE('',#3437,#3412,#2273,.T.);
#4313=EDGE_CURVE('',#3439,#3410,#2274,.T.);
#4314=EDGE_CURVE('',#3409,#3440,#2275,.T.);
#4315=EDGE_CURVE('',#3434,#3366,#2276,.T.);
#4316=EDGE_CURVE('',#3365,#3435,#2277,.T.);
#4317=EDGE_CURVE('',#3436,#3364,#2278,.T.);
#4318=EDGE_CURVE('',#3369,#3441,#2279,.T.);
#4319=EDGE_CURVE('',#3441,#3441,#1614,.T.);
#4320=EDGE_CURVE('',#3419,#3442,#2280,.T.);
#4321=EDGE_CURVE('',#3442,#3442,#1615,.T.);
#4322=EDGE_CURVE('',#3418,#3443,#2281,.T.);
#4323=EDGE_CURVE('',#3443,#3443,#1616,.T.);
#4324=EDGE_CURVE('',#3370,#3444,#2282,.T.);
#4325=EDGE_CURVE('',#3444,#3444,#1617,.T.);
#4326=EDGE_CURVE('',#3445,#3446,#1618,.T.);
#4327=EDGE_CURVE('',#3446,#3447,#2283,.T.);
#4328=EDGE_CURVE('',#3447,#3448,#1619,.T.);
#4329=EDGE_CURVE('',#3448,#3445,#2284,.T.);
#4330=EDGE_CURVE('',#3449,#3450,#1620,.T.);
#4331=EDGE_CURVE('',#3450,#3448,#1621,.T.);
#4332=EDGE_CURVE('',#3447,#3449,#1622,.T.);
#4333=EDGE_CURVE('',#3451,#3452,#1623,.T.);
#4334=EDGE_CURVE('',#3452,#3450,#2285,.T.);
#4335=EDGE_CURVE('',#3449,#3451,#2286,.T.);
#4336=EDGE_CURVE('',#3453,#3454,#1624,.T.);
#4337=EDGE_CURVE('',#3454,#3452,#1625,.T.);
#4338=EDGE_CURVE('',#3451,#3453,#1626,.T.);
#4339=EDGE_CURVE('',#3455,#3456,#1627,.T.);
#4340=EDGE_CURVE('',#3456,#3454,#2287,.T.);
#4341=EDGE_CURVE('',#3453,#3455,#2288,.T.);
#4342=EDGE_CURVE('',#3399,#3457,#1628,.T.);
#4343=EDGE_CURVE('',#3457,#3456,#1629,.T.);
#4344=EDGE_CURVE('',#3455,#3399,#1630,.T.);
#4345=EDGE_CURVE('',#3398,#3458,#1631,.T.);
#4346=EDGE_CURVE('',#3458,#3457,#2289,.T.);
#4347=EDGE_CURVE('',#3459,#3460,#1632,.T.);
#4348=EDGE_CURVE('',#3460,#3458,#1633,.T.);
#4349=EDGE_CURVE('',#3398,#3459,#1634,.T.);
#4350=EDGE_CURVE('',#3461,#3462,#1635,.T.);
#4351=EDGE_CURVE('',#3462,#3460,#2290,.T.);
#4352=EDGE_CURVE('',#3459,#3461,#2291,.T.);
#4353=EDGE_CURVE('',#3429,#3463,#1636,.T.);
#4354=EDGE_CURVE('',#3463,#3462,#1637,.T.);
#4355=EDGE_CURVE('',#3461,#3429,#1638,.T.);
#4356=EDGE_CURVE('',#3428,#3464,#1639,.T.);
#4357=EDGE_CURVE('',#3464,#3463,#2292,.T.);
#4358=EDGE_CURVE('',#3445,#3464,#1640,.T.);
#4359=EDGE_CURVE('',#3428,#3446,#1641,.T.);
#4360=EDGE_CURVE('',#3355,#3455,#2293,.T.);
#4361=EDGE_CURVE('',#3356,#3453,#2294,.T.);
#4362=EDGE_CURVE('',#3357,#3451,#2295,.T.);
#4363=EDGE_CURVE('',#3358,#3449,#2296,.T.);
#4364=EDGE_CURVE('',#3359,#3447,#2297,.T.);
#4365=EDGE_CURVE('',#3360,#3446,#2298,.T.);
#4366=EDGE_CURVE('',#3416,#3461,#2299,.T.);
#4367=EDGE_CURVE('',#3417,#3459,#2300,.T.);
#5643=ORIENTED_EDGE('',*,*,#4189,.T.);
#5644=ORIENTED_EDGE('',*,*,#4190,.F.);
#5645=ORIENTED_EDGE('',*,*,#4191,.F.);
#5646=ORIENTED_EDGE('',*,*,#4192,.F.);
#5647=ORIENTED_EDGE('',*,*,#4193,.F.);
#5648=ORIENTED_EDGE('',*,*,#4194,.F.);
#5649=ORIENTED_EDGE('',*,*,#4195,.T.);
#5650=ORIENTED_EDGE('',*,*,#4196,.F.);
#5651=ORIENTED_EDGE('',*,*,#4197,.F.);
#5652=ORIENTED_EDGE('',*,*,#4198,.F.);
#5653=ORIENTED_EDGE('',*,*,#4199,.T.);
#5654=ORIENTED_EDGE('',*,*,#4200,.T.);
#5655=ORIENTED_EDGE('',*,*,#4201,.T.);
#5656=ORIENTED_EDGE('',*,*,#4202,.T.);
#5657=ORIENTED_EDGE('',*,*,#4203,.T.);
#5658=ORIENTED_EDGE('',*,*,#4204,.T.);
#5659=ORIENTED_EDGE('',*,*,#4205,.T.);
#5660=ORIENTED_EDGE('',*,*,#4206,.T.);
#5661=ORIENTED_EDGE('',*,*,#4207,.T.);
#5662=ORIENTED_EDGE('',*,*,#4208,.T.);
#5663=ORIENTED_EDGE('',*,*,#4209,.T.);
#5664=ORIENTED_EDGE('',*,*,#4210,.T.);
#5665=ORIENTED_EDGE('',*,*,#4211,.T.);
#5666=ORIENTED_EDGE('',*,*,#4212,.T.);
#5667=ORIENTED_EDGE('',*,*,#4213,.T.);
#5668=ORIENTED_EDGE('',*,*,#4208,.F.);
#5669=ORIENTED_EDGE('',*,*,#4214,.T.);
#5670=ORIENTED_EDGE('',*,*,#4215,.T.);
#5671=ORIENTED_EDGE('',*,*,#4216,.T.);
#5672=ORIENTED_EDGE('',*,*,#4217,.T.);
#5673=ORIENTED_EDGE('',*,*,#4218,.T.);
#5674=ORIENTED_EDGE('',*,*,#4219,.T.);
#5675=ORIENTED_EDGE('',*,*,#4217,.F.);
#5676=ORIENTED_EDGE('',*,*,#4220,.T.);
#5677=ORIENTED_EDGE('',*,*,#4221,.T.);
#5678=ORIENTED_EDGE('',*,*,#4222,.T.);
#5679=ORIENTED_EDGE('',*,*,#4223,.T.);
#5680=ORIENTED_EDGE('',*,*,#4224,.T.);
#5681=ORIENTED_EDGE('',*,*,#4221,.F.);
#5682=ORIENTED_EDGE('',*,*,#4223,.F.);
#5683=ORIENTED_EDGE('',*,*,#4225,.T.);
#5684=ORIENTED_EDGE('',*,*,#4212,.F.);
#5685=ORIENTED_EDGE('',*,*,#4226,.T.);
#5686=ORIENTED_EDGE('',*,*,#4209,.F.);
#5687=ORIENTED_EDGE('',*,*,#4227,.F.);
#5688=ORIENTED_EDGE('',*,*,#4228,.F.);
#5689=ORIENTED_EDGE('',*,*,#4229,.T.);
#5690=ORIENTED_EDGE('',*,*,#4213,.F.);
#5691=ORIENTED_EDGE('',*,*,#4230,.F.);
#5692=ORIENTED_EDGE('',*,*,#4231,.F.);
#5693=ORIENTED_EDGE('',*,*,#4227,.T.);
#5694=ORIENTED_EDGE('',*,*,#4225,.F.);
#5695=ORIENTED_EDGE('',*,*,#4232,.T.);
#5696=ORIENTED_EDGE('',*,*,#4233,.T.);
#5697=ORIENTED_EDGE('',*,*,#4234,.T.);
#5698=ORIENTED_EDGE('',*,*,#4230,.T.);
#5699=ORIENTED_EDGE('',*,*,#4222,.F.);
#5700=ORIENTED_EDGE('',*,*,#4235,.F.);
#5701=ORIENTED_EDGE('',*,*,#4236,.T.);
#5702=ORIENTED_EDGE('',*,*,#4232,.F.);
#5703=ORIENTED_EDGE('',*,*,#4237,.T.);
#5704=ORIENTED_EDGE('',*,*,#4235,.T.);
#5705=ORIENTED_EDGE('',*,*,#4220,.F.);
#5706=ORIENTED_EDGE('',*,*,#4238,.F.);
#5707=ORIENTED_EDGE('',*,*,#4239,.F.);
#5708=ORIENTED_EDGE('',*,*,#4240,.T.);
#5709=ORIENTED_EDGE('',*,*,#4241,.F.);
#5710=ORIENTED_EDGE('',*,*,#4242,.F.);
#5711=ORIENTED_EDGE('',*,*,#4210,.F.);
#5712=ORIENTED_EDGE('',*,*,#4243,.T.);
#5713=ORIENTED_EDGE('',*,*,#4215,.F.);
#5714=ORIENTED_EDGE('',*,*,#4244,.T.);
#5715=ORIENTED_EDGE('',*,*,#4216,.F.);
#5716=ORIENTED_EDGE('',*,*,#4245,.F.);
#5717=ORIENTED_EDGE('',*,*,#4246,.F.);
#5718=ORIENTED_EDGE('',*,*,#4238,.T.);
#5719=ORIENTED_EDGE('',*,*,#4211,.F.);
#5720=ORIENTED_EDGE('',*,*,#4244,.F.);
#5721=ORIENTED_EDGE('',*,*,#4218,.F.);
#5722=ORIENTED_EDGE('',*,*,#4219,.F.);
#5723=ORIENTED_EDGE('',*,*,#4224,.F.);
#5724=ORIENTED_EDGE('',*,*,#4226,.F.);
#5725=ORIENTED_EDGE('',*,*,#4214,.F.);
#5726=ORIENTED_EDGE('',*,*,#4234,.F.);
#5727=ORIENTED_EDGE('',*,*,#4247,.T.);
#5728=ORIENTED_EDGE('',*,*,#4248,.T.);
#5729=ORIENTED_EDGE('',*,*,#4249,.F.);
#5730=ORIENTED_EDGE('',*,*,#4250,.F.);
#5731=ORIENTED_EDGE('',*,*,#4190,.T.);
#5732=ORIENTED_EDGE('',*,*,#4251,.T.);
#5733=ORIENTED_EDGE('',*,*,#4252,.T.);
#5734=ORIENTED_EDGE('',*,*,#4253,.T.);
#5735=ORIENTED_EDGE('',*,*,#4254,.T.);
#5736=ORIENTED_EDGE('',*,*,#4239,.T.);
#5737=ORIENTED_EDGE('',*,*,#4246,.T.);
#5738=ORIENTED_EDGE('',*,*,#4255,.T.);
#5739=ORIENTED_EDGE('',*,*,#4228,.T.);
#5740=ORIENTED_EDGE('',*,*,#4231,.T.);
#5741=ORIENTED_EDGE('',*,*,#4256,.F.);
#5742=ORIENTED_EDGE('',*,*,#4257,.T.);
#5743=ORIENTED_EDGE('',*,*,#4237,.F.);
#5744=ORIENTED_EDGE('',*,*,#4257,.F.);
#5745=ORIENTED_EDGE('',*,*,#4243,.F.);
#5746=ORIENTED_EDGE('',*,*,#4229,.F.);
#5747=ORIENTED_EDGE('',*,*,#4255,.F.);
#5748=ORIENTED_EDGE('',*,*,#4245,.T.);
#5749=ORIENTED_EDGE('',*,*,#4256,.T.);
#5750=ORIENTED_EDGE('',*,*,#4189,.F.);
#5751=ORIENTED_EDGE('',*,*,#4258,.F.);
#5752=ORIENTED_EDGE('',*,*,#4259,.F.);
#5753=ORIENTED_EDGE('',*,*,#4251,.F.);
#5754=ORIENTED_EDGE('',*,*,#4253,.F.);
#5755=ORIENTED_EDGE('',*,*,#4260,.T.);
#5756=ORIENTED_EDGE('',*,*,#4261,.F.);
#5757=ORIENTED_EDGE('',*,*,#4262,.F.);
#5758=ORIENTED_EDGE('',*,*,#4252,.F.);
#5759=ORIENTED_EDGE('',*,*,#4259,.T.);
#5760=ORIENTED_EDGE('',*,*,#4263,.F.);
#5761=ORIENTED_EDGE('',*,*,#4264,.F.);
#5762=ORIENTED_EDGE('',*,*,#4260,.F.);
#5763=ORIENTED_EDGE('',*,*,#4254,.F.);
#5764=ORIENTED_EDGE('',*,*,#4262,.T.);
#5765=ORIENTED_EDGE('',*,*,#4265,.F.);
#5766=ORIENTED_EDGE('',*,*,#4240,.F.);
#5767=ORIENTED_EDGE('',*,*,#4242,.T.);
#5768=ORIENTED_EDGE('',*,*,#4266,.T.);
#5769=ORIENTED_EDGE('',*,*,#4267,.T.);
#5770=ORIENTED_EDGE('',*,*,#4268,.T.);
#5771=ORIENTED_EDGE('',*,*,#4269,.T.);
#5772=ORIENTED_EDGE('',*,*,#4270,.T.);
#5773=ORIENTED_EDGE('',*,*,#4271,.T.);
#5774=ORIENTED_EDGE('',*,*,#4272,.T.);
#5775=ORIENTED_EDGE('',*,*,#4273,.F.);
#5776=ORIENTED_EDGE('',*,*,#4274,.F.);
#5777=ORIENTED_EDGE('',*,*,#4275,.F.);
#5778=ORIENTED_EDGE('',*,*,#4276,.F.);
#5779=ORIENTED_EDGE('',*,*,#4247,.F.);
#5780=ORIENTED_EDGE('',*,*,#4233,.F.);
#5781=ORIENTED_EDGE('',*,*,#4236,.F.);
#5782=ORIENTED_EDGE('',*,*,#4277,.T.);
#5783=ORIENTED_EDGE('',*,*,#4278,.T.);
#5784=ORIENTED_EDGE('',*,*,#4279,.F.);
#5785=ORIENTED_EDGE('',*,*,#4280,.F.);
#5786=ORIENTED_EDGE('',*,*,#4281,.F.);
#5787=ORIENTED_EDGE('',*,*,#4282,.T.);
#5788=ORIENTED_EDGE('',*,*,#4283,.F.);
#5789=ORIENTED_EDGE('',*,*,#4282,.F.);
#5790=ORIENTED_EDGE('',*,*,#4284,.F.);
#5791=ORIENTED_EDGE('',*,*,#4272,.F.);
#5792=ORIENTED_EDGE('',*,*,#4285,.F.);
#5793=ORIENTED_EDGE('',*,*,#4199,.F.);
#5794=ORIENTED_EDGE('',*,*,#4286,.F.);
#5795=ORIENTED_EDGE('',*,*,#4287,.T.);
#5796=ORIENTED_EDGE('',*,*,#4288,.F.);
#5797=ORIENTED_EDGE('',*,*,#4287,.F.);
#5798=ORIENTED_EDGE('',*,*,#4289,.F.);
#5799=ORIENTED_EDGE('',*,*,#4290,.T.);
#5800=ORIENTED_EDGE('',*,*,#4291,.F.);
#5801=ORIENTED_EDGE('',*,*,#4290,.F.);
#5802=ORIENTED_EDGE('',*,*,#4292,.F.);
#5803=ORIENTED_EDGE('',*,*,#4280,.T.);
#5804=ORIENTED_EDGE('',*,*,#4284,.T.);
#5805=ORIENTED_EDGE('',*,*,#4281,.T.);
#5806=ORIENTED_EDGE('',*,*,#4292,.T.);
#5807=ORIENTED_EDGE('',*,*,#4289,.T.);
#5808=ORIENTED_EDGE('',*,*,#4286,.T.);
#5809=ORIENTED_EDGE('',*,*,#4198,.T.);
#5810=ORIENTED_EDGE('',*,*,#4293,.T.);
#5811=ORIENTED_EDGE('',*,*,#4294,.F.);
#5812=ORIENTED_EDGE('',*,*,#4295,.F.);
#5813=ORIENTED_EDGE('',*,*,#4273,.T.);
#5814=ORIENTED_EDGE('',*,*,#4264,.T.);
#5815=ORIENTED_EDGE('',*,*,#4296,.T.);
#5816=ORIENTED_EDGE('',*,*,#4297,.T.);
#5817=ORIENTED_EDGE('',*,*,#4298,.T.);
#5818=ORIENTED_EDGE('',*,*,#4266,.F.);
#5819=ORIENTED_EDGE('',*,*,#4241,.T.);
#5820=ORIENTED_EDGE('',*,*,#4265,.T.);
#5821=ORIENTED_EDGE('',*,*,#4261,.T.);
#5822=ORIENTED_EDGE('',*,*,#4299,.T.);
#5823=ORIENTED_EDGE('',*,*,#4300,.F.);
#5824=ORIENTED_EDGE('',*,*,#4301,.T.);
#5825=ORIENTED_EDGE('',*,*,#4302,.F.);
#5826=ORIENTED_EDGE('',*,*,#4303,.T.);
#5827=ORIENTED_EDGE('',*,*,#4304,.F.);
#5828=ORIENTED_EDGE('',*,*,#4305,.F.);
#5829=ORIENTED_EDGE('',*,*,#4306,.T.);
#5830=ORIENTED_EDGE('',*,*,#4307,.F.);
#5831=ORIENTED_EDGE('',*,*,#4308,.T.);
#5832=ORIENTED_EDGE('',*,*,#4297,.F.);
#5833=ORIENTED_EDGE('',*,*,#4309,.T.);
#5834=ORIENTED_EDGE('',*,*,#4204,.F.);
#5835=ORIENTED_EDGE('',*,*,#4310,.T.);
#5836=ORIENTED_EDGE('',*,*,#4300,.T.);
#5837=ORIENTED_EDGE('',*,*,#4311,.T.);
#5838=ORIENTED_EDGE('',*,*,#4305,.T.);
#5839=ORIENTED_EDGE('',*,*,#4312,.T.);
#5840=ORIENTED_EDGE('',*,*,#4270,.F.);
#5841=ORIENTED_EDGE('',*,*,#4313,.T.);
#5842=ORIENTED_EDGE('',*,*,#4268,.F.);
#5843=ORIENTED_EDGE('',*,*,#4314,.T.);
#5844=ORIENTED_EDGE('',*,*,#4307,.T.);
#5845=ORIENTED_EDGE('',*,*,#4315,.T.);
#5846=ORIENTED_EDGE('',*,*,#4202,.F.);
#5847=ORIENTED_EDGE('',*,*,#4316,.T.);
#5848=ORIENTED_EDGE('',*,*,#4302,.T.);
#5849=ORIENTED_EDGE('',*,*,#4283,.T.);
#5850=ORIENTED_EDGE('',*,*,#4271,.F.);
#5851=ORIENTED_EDGE('',*,*,#4312,.F.);
#5852=ORIENTED_EDGE('',*,*,#4304,.T.);
#5853=ORIENTED_EDGE('',*,*,#4317,.T.);
#5854=ORIENTED_EDGE('',*,*,#4200,.F.);
#5855=ORIENTED_EDGE('',*,*,#4285,.T.);
#5856=ORIENTED_EDGE('',*,*,#4288,.T.);
#5857=ORIENTED_EDGE('',*,*,#4291,.T.);
#5858=ORIENTED_EDGE('',*,*,#4279,.T.);
#5859=ORIENTED_EDGE('',*,*,#4301,.F.);
#5860=ORIENTED_EDGE('',*,*,#4310,.F.);
#5861=ORIENTED_EDGE('',*,*,#4203,.F.);
#5862=ORIENTED_EDGE('',*,*,#4315,.F.);
#5863=ORIENTED_EDGE('',*,*,#4298,.F.);
#5864=ORIENTED_EDGE('',*,*,#4308,.F.);
#5865=ORIENTED_EDGE('',*,*,#4314,.F.);
#5866=ORIENTED_EDGE('',*,*,#4267,.F.);
#5867=ORIENTED_EDGE('',*,*,#4313,.F.);
#5868=ORIENTED_EDGE('',*,*,#4306,.F.);
#5869=ORIENTED_EDGE('',*,*,#4311,.F.);
#5870=ORIENTED_EDGE('',*,*,#4269,.F.);
#5871=ORIENTED_EDGE('',*,*,#4258,.T.);
#5872=ORIENTED_EDGE('',*,*,#4205,.F.);
#5873=ORIENTED_EDGE('',*,*,#4309,.F.);
#5874=ORIENTED_EDGE('',*,*,#4299,.F.);
#5875=ORIENTED_EDGE('',*,*,#4296,.F.);
#5876=ORIENTED_EDGE('',*,*,#4263,.T.);
#5877=ORIENTED_EDGE('',*,*,#4201,.F.);
#5878=ORIENTED_EDGE('',*,*,#4317,.F.);
#5879=ORIENTED_EDGE('',*,*,#4303,.F.);
#5880=ORIENTED_EDGE('',*,*,#4316,.F.);
#5881=ORIENTED_EDGE('',*,*,#4206,.F.);
#5882=ORIENTED_EDGE('',*,*,#4318,.T.);
#5883=ORIENTED_EDGE('',*,*,#4319,.T.);
#5884=ORIENTED_EDGE('',*,*,#4318,.F.);
#5885=ORIENTED_EDGE('',*,*,#4319,.F.);
#5886=ORIENTED_EDGE('',*,*,#4278,.F.);
#5887=ORIENTED_EDGE('',*,*,#4320,.T.);
#5888=ORIENTED_EDGE('',*,*,#4321,.T.);
#5889=ORIENTED_EDGE('',*,*,#4320,.F.);
#5890=ORIENTED_EDGE('',*,*,#4321,.F.);
#5891=ORIENTED_EDGE('',*,*,#4277,.F.);
#5892=ORIENTED_EDGE('',*,*,#4322,.T.);
#5893=ORIENTED_EDGE('',*,*,#4323,.T.);
#5894=ORIENTED_EDGE('',*,*,#4322,.F.);
#5895=ORIENTED_EDGE('',*,*,#4323,.F.);
#5896=ORIENTED_EDGE('',*,*,#4207,.F.);
#5897=ORIENTED_EDGE('',*,*,#4324,.T.);
#5898=ORIENTED_EDGE('',*,*,#4325,.T.);
#5899=ORIENTED_EDGE('',*,*,#4324,.F.);
#5900=ORIENTED_EDGE('',*,*,#4325,.F.);
#5901=ORIENTED_EDGE('',*,*,#4326,.T.);
#5902=ORIENTED_EDGE('',*,*,#4327,.T.);
#5903=ORIENTED_EDGE('',*,*,#4328,.T.);
#5904=ORIENTED_EDGE('',*,*,#4329,.T.);
#5905=ORIENTED_EDGE('',*,*,#4330,.T.);
#5906=ORIENTED_EDGE('',*,*,#4331,.T.);
#5907=ORIENTED_EDGE('',*,*,#4328,.F.);
#5908=ORIENTED_EDGE('',*,*,#4332,.T.);
#5909=ORIENTED_EDGE('',*,*,#4333,.T.);
#5910=ORIENTED_EDGE('',*,*,#4334,.T.);
#5911=ORIENTED_EDGE('',*,*,#4330,.F.);
#5912=ORIENTED_EDGE('',*,*,#4335,.T.);
#5913=ORIENTED_EDGE('',*,*,#4336,.T.);
#5914=ORIENTED_EDGE('',*,*,#4337,.T.);
#5915=ORIENTED_EDGE('',*,*,#4333,.F.);
#5916=ORIENTED_EDGE('',*,*,#4338,.T.);
#5917=ORIENTED_EDGE('',*,*,#4339,.T.);
#5918=ORIENTED_EDGE('',*,*,#4340,.T.);
#5919=ORIENTED_EDGE('',*,*,#4336,.F.);
#5920=ORIENTED_EDGE('',*,*,#4341,.T.);
#5921=ORIENTED_EDGE('',*,*,#4342,.T.);
#5922=ORIENTED_EDGE('',*,*,#4343,.T.);
#5923=ORIENTED_EDGE('',*,*,#4339,.F.);
#5924=ORIENTED_EDGE('',*,*,#4344,.T.);
#5925=ORIENTED_EDGE('',*,*,#4345,.T.);
#5926=ORIENTED_EDGE('',*,*,#4346,.T.);
#5927=ORIENTED_EDGE('',*,*,#4342,.F.);
#5928=ORIENTED_EDGE('',*,*,#4249,.T.);
#5929=ORIENTED_EDGE('',*,*,#4347,.T.);
#5930=ORIENTED_EDGE('',*,*,#4348,.T.);
#5931=ORIENTED_EDGE('',*,*,#4345,.F.);
#5932=ORIENTED_EDGE('',*,*,#4349,.T.);
#5933=ORIENTED_EDGE('',*,*,#4350,.T.);
#5934=ORIENTED_EDGE('',*,*,#4351,.T.);
#5935=ORIENTED_EDGE('',*,*,#4347,.F.);
#5936=ORIENTED_EDGE('',*,*,#4352,.T.);
#5937=ORIENTED_EDGE('',*,*,#4353,.T.);
#5938=ORIENTED_EDGE('',*,*,#4354,.T.);
#5939=ORIENTED_EDGE('',*,*,#4350,.F.);
#5940=ORIENTED_EDGE('',*,*,#4355,.T.);
#5941=ORIENTED_EDGE('',*,*,#4356,.T.);
#5942=ORIENTED_EDGE('',*,*,#4357,.T.);
#5943=ORIENTED_EDGE('',*,*,#4353,.F.);
#5944=ORIENTED_EDGE('',*,*,#4294,.T.);
#5945=ORIENTED_EDGE('',*,*,#4326,.F.);
#5946=ORIENTED_EDGE('',*,*,#4358,.T.);
#5947=ORIENTED_EDGE('',*,*,#4356,.F.);
#5948=ORIENTED_EDGE('',*,*,#4359,.T.);
#5949=ORIENTED_EDGE('',*,*,#4344,.F.);
#5950=ORIENTED_EDGE('',*,*,#4360,.F.);
#5951=ORIENTED_EDGE('',*,*,#4191,.T.);
#5952=ORIENTED_EDGE('',*,*,#4250,.T.);
#5953=ORIENTED_EDGE('',*,*,#4341,.F.);
#5954=ORIENTED_EDGE('',*,*,#4361,.F.);
#5955=ORIENTED_EDGE('',*,*,#4192,.T.);
#5956=ORIENTED_EDGE('',*,*,#4360,.T.);
#5957=ORIENTED_EDGE('',*,*,#4338,.F.);
#5958=ORIENTED_EDGE('',*,*,#4362,.F.);
#5959=ORIENTED_EDGE('',*,*,#4193,.T.);
#5960=ORIENTED_EDGE('',*,*,#4361,.T.);
#5961=ORIENTED_EDGE('',*,*,#4335,.F.);
#5962=ORIENTED_EDGE('',*,*,#4363,.F.);
#5963=ORIENTED_EDGE('',*,*,#4194,.T.);
#5964=ORIENTED_EDGE('',*,*,#4362,.T.);
#5965=ORIENTED_EDGE('',*,*,#4332,.F.);
#5966=ORIENTED_EDGE('',*,*,#4364,.F.);
#5967=ORIENTED_EDGE('',*,*,#4195,.F.);
#5968=ORIENTED_EDGE('',*,*,#4363,.T.);
#5969=ORIENTED_EDGE('',*,*,#4327,.F.);
#5970=ORIENTED_EDGE('',*,*,#4365,.F.);
#5971=ORIENTED_EDGE('',*,*,#4196,.T.);
#5972=ORIENTED_EDGE('',*,*,#4364,.T.);
#5973=ORIENTED_EDGE('',*,*,#4329,.F.);
#5974=ORIENTED_EDGE('',*,*,#4331,.F.);
#5975=ORIENTED_EDGE('',*,*,#4334,.F.);
#5976=ORIENTED_EDGE('',*,*,#4337,.F.);
#5977=ORIENTED_EDGE('',*,*,#4340,.F.);
#5978=ORIENTED_EDGE('',*,*,#4343,.F.);
#5979=ORIENTED_EDGE('',*,*,#4346,.F.);
#5980=ORIENTED_EDGE('',*,*,#4348,.F.);
#5981=ORIENTED_EDGE('',*,*,#4351,.F.);
#5982=ORIENTED_EDGE('',*,*,#4354,.F.);
#5983=ORIENTED_EDGE('',*,*,#4357,.F.);
#5984=ORIENTED_EDGE('',*,*,#4358,.F.);
#5985=ORIENTED_EDGE('',*,*,#4359,.F.);
#5986=ORIENTED_EDGE('',*,*,#4293,.F.);
#5987=ORIENTED_EDGE('',*,*,#4197,.T.);
#5988=ORIENTED_EDGE('',*,*,#4365,.T.);
#5989=ORIENTED_EDGE('',*,*,#4355,.F.);
#5990=ORIENTED_EDGE('',*,*,#4366,.F.);
#5991=ORIENTED_EDGE('',*,*,#4274,.T.);
#5992=ORIENTED_EDGE('',*,*,#4295,.T.);
#5993=ORIENTED_EDGE('',*,*,#4352,.F.);
#5994=ORIENTED_EDGE('',*,*,#4367,.F.);
#5995=ORIENTED_EDGE('',*,*,#4275,.T.);
#5996=ORIENTED_EDGE('',*,*,#4366,.T.);
#5997=ORIENTED_EDGE('',*,*,#4349,.F.);
#5998=ORIENTED_EDGE('',*,*,#4248,.F.);
#5999=ORIENTED_EDGE('',*,*,#4276,.T.);
#6000=ORIENTED_EDGE('',*,*,#4367,.T.);
#7485=CYLINDRICAL_SURFACE('',#8477,1.);
#7486=CYLINDRICAL_SURFACE('',#8483,1.);
#7487=CYLINDRICAL_SURFACE('',#8485,1.);
#7488=CYLINDRICAL_SURFACE('',#8489,2.);
#7489=CYLINDRICAL_SURFACE('',#8492,2.);
#7490=CYLINDRICAL_SURFACE('',#8497,1.);
#7491=CYLINDRICAL_SURFACE('',#8498,2.);
#7492=CYLINDRICAL_SURFACE('',#8504,4.);
#7493=CYLINDRICAL_SURFACE('',#8509,0.999999999999999);
#7494=CYLINDRICAL_SURFACE('',#8511,1.);
#7495=CYLINDRICAL_SURFACE('',#8520,2.);
#7496=CYLINDRICAL_SURFACE('',#8525,2.);
#7497=CYLINDRICAL_SURFACE('',#8540,3.);
#7498=CYLINDRICAL_SURFACE('',#8542,3.5);
#7499=CYLINDRICAL_SURFACE('',#8543,3.5);
#7500=CYLINDRICAL_SURFACE('',#8544,3.5);
#7501=CYLINDRICAL_SURFACE('',#8545,3.5);
#7502=CYLINDRICAL_SURFACE('',#8547,1.5);
#7503=CYLINDRICAL_SURFACE('',#8550,1.5);
#7504=CYLINDRICAL_SURFACE('',#8553,1.5);
#7505=CYLINDRICAL_SURFACE('',#8556,1.5);
#7506=CYLINDRICAL_SURFACE('',#8559,1.);
#7507=CYLINDRICAL_SURFACE('',#8566,1.);
#7508=CYLINDRICAL_SURFACE('',#8571,1.);
#7509=CYLINDRICAL_SURFACE('',#8576,1.);
#7510=CYLINDRICAL_SURFACE('',#8581,1.);
#7511=CYLINDRICAL_SURFACE('',#8586,1.);
#7512=CYLINDRICAL_SURFACE('',#8590,2.);
#7513=CYLINDRICAL_SURFACE('',#8592,1.99999999999999);
#7514=CYLINDRICAL_SURFACE('',#8594,0.999999999999996);
#7515=CYLINDRICAL_SURFACE('',#8597,2.00000000000001);
#7516=CYLINDRICAL_SURFACE('',#8598,2.);
#7517=CYLINDRICAL_SURFACE('',#8600,2.);
#7739=ADVANCED_FACE('',(#577,#142,#143),#330,.F.);
#7740=ADVANCED_FACE('',(#578),#180,.F.);
#7741=ADVANCED_FACE('',(#579),#7485,.T.);
#7742=ADVANCED_FACE('',(#580),#181,.F.);
#7743=ADVANCED_FACE('',(#581),#7486,.T.);
#7744=ADVANCED_FACE('',(#582),#7487,.T.);
#7745=ADVANCED_FACE('',(#583),#182,.F.);
#7746=ADVANCED_FACE('',(#584),#7488,.T.);
#7747=ADVANCED_FACE('',(#585),#331,.T.);
#7748=ADVANCED_FACE('',(#586),#7489,.T.);
#7749=ADVANCED_FACE('',(#587,#144),#332,.T.);
#7750=ADVANCED_FACE('',(#588),#333,.F.);
#7751=ADVANCED_FACE('',(#589),#7490,.T.);
#7752=ADVANCED_FACE('',(#590),#7491,.T.);
#7753=ADVANCED_FACE('',(#591),#334,.T.);
#7754=ADVANCED_FACE('',(#592),#335,.T.);
#7755=ADVANCED_FACE('',(#593),#7492,.F.);
#7756=ADVANCED_FACE('',(#594,#145),#336,.T.);
#7757=ADVANCED_FACE('',(#595),#337,.F.);
#7758=ADVANCED_FACE('',(#596),#338,.F.);
#7759=ADVANCED_FACE('',(#597),#7493,.F.);
#7760=ADVANCED_FACE('',(#598),#7494,.F.);
#7761=ADVANCED_FACE('',(#599,#146,#147),#339,.F.);
#7762=ADVANCED_FACE('',(#600),#7495,.F.);
#7763=ADVANCED_FACE('',(#601),#340,.F.);
#7764=ADVANCED_FACE('',(#602),#341,.F.);
#7765=ADVANCED_FACE('',(#603),#7496,.F.);
#7766=ADVANCED_FACE('',(#604),#342,.F.);
#7767=ADVANCED_FACE('',(#605),#343,.T.);
#7768=ADVANCED_FACE('',(#606),#344,.F.);
#7769=ADVANCED_FACE('',(#607),#345,.F.);
#7770=ADVANCED_FACE('',(#608),#346,.F.);
#7771=ADVANCED_FACE('',(#609),#347,.F.);
#7772=ADVANCED_FACE('',(#610),#348,.F.);
#7773=ADVANCED_FACE('',(#611),#7497,.T.);
#7774=ADVANCED_FACE('',(#612),#349,.F.);
#7775=ADVANCED_FACE('',(#613),#7498,.T.);
#7776=ADVANCED_FACE('',(#614),#7499,.T.);
#7777=ADVANCED_FACE('',(#615),#7500,.T.);
#7778=ADVANCED_FACE('',(#616),#7501,.T.);
#7779=ADVANCED_FACE('',(#617),#350,.F.);
#7780=ADVANCED_FACE('',(#618),#7502,.F.);
#7781=ADVANCED_FACE('',(#619),#351,.T.);
#7782=ADVANCED_FACE('',(#620),#7503,.F.);
#7783=ADVANCED_FACE('',(#621),#352,.T.);
#7784=ADVANCED_FACE('',(#622),#7504,.F.);
#7785=ADVANCED_FACE('',(#623),#353,.T.);
#7786=ADVANCED_FACE('',(#624),#7505,.F.);
#7787=ADVANCED_FACE('',(#625),#354,.T.);
#7788=ADVANCED_FACE('',(#626),#7506,.T.);
#7789=ADVANCED_FACE('',(#627),#219,.T.);
#7790=ADVANCED_FACE('',(#628),#7507,.T.);
#7791=ADVANCED_FACE('',(#629),#183,.F.);
#7792=ADVANCED_FACE('',(#630),#7508,.T.);
#7793=ADVANCED_FACE('',(#631),#184,.F.);
#7794=ADVANCED_FACE('',(#632),#7509,.T.);
#7795=ADVANCED_FACE('',(#633),#185,.F.);
#7796=ADVANCED_FACE('',(#634),#7510,.T.);
#7797=ADVANCED_FACE('',(#635),#186,.F.);
#7798=ADVANCED_FACE('',(#636),#7511,.T.);
#7799=ADVANCED_FACE('',(#637),#187,.F.);
#7800=ADVANCED_FACE('',(#638),#7512,.T.);
#7801=ADVANCED_FACE('',(#639),#355,.T.);
#7802=ADVANCED_FACE('',(#640),#7513,.T.);
#7803=ADVANCED_FACE('',(#641),#356,.T.);
#7804=ADVANCED_FACE('',(#642),#7514,.F.);
#7805=ADVANCED_FACE('',(#643),#357,.T.);
#7806=ADVANCED_FACE('',(#644),#358,.T.);
#7807=ADVANCED_FACE('',(#645),#7515,.T.);
#7808=ADVANCED_FACE('',(#646),#7516,.T.);
#7809=ADVANCED_FACE('',(#647),#359,.T.);
#7810=ADVANCED_FACE('',(#648),#7517,.T.);
#8116=CLOSED_SHELL('',(#7739,#7740,#7741,#7742,#7743,#7744,#7745,#7746,
#7747,#7748,#7749,#7750,#7751,#7752,#7753,#7754,#7755,#7756,#7757,#7758,
#7759,#7760,#7761,#7762,#7763,#7764,#7765,#7766,#7767,#7768,#7769,#7770,
#7771,#7772,#7773,#7774,#7775,#7776,#7777,#7778,#7779,#7780,#7781,#7782,
#7783,#7784,#7785,#7786,#7787,#7788,#7789,#7790,#7791,#7792,#7793,#7794,
#7795,#7796,#7797,#7798,#7799,#7800,#7801,#7802,#7803,#7804,#7805,#7806,
#7807,#7808,#7809,#7810));
#8462=AXIS2_PLACEMENT_3D('',#12392,#9830,#9831);
#8463=AXIS2_PLACEMENT_3D('',#12393,#9832,#9833);
#8464=AXIS2_PLACEMENT_3D('',#12400,#9836,#9837);
#8465=AXIS2_PLACEMENT_3D('',#12404,#9839,#9840);
#8466=AXIS2_PLACEMENT_3D('',#12408,#9842,#9843);
#8467=AXIS2_PLACEMENT_3D('',#12412,#9845,#9846);
#8468=AXIS2_PLACEMENT_3D('',#12422,#9851,#9852);
#8469=AXIS2_PLACEMENT_3D('',#12424,#9853,#9854);
#8470=AXIS2_PLACEMENT_3D('',#12427,#9856,#9857);
#8471=AXIS2_PLACEMENT_3D('',#12429,#9858,#9859);
#8472=AXIS2_PLACEMENT_3D('',#12431,#9860,#9861);
#8473=AXIS2_PLACEMENT_3D('',#12443,#9862,#9863);
#8474=AXIS2_PLACEMENT_3D('',#12445,#9864,#9865);
#8475=AXIS2_PLACEMENT_3D('',#12447,#9866,#9867);
#8476=AXIS2_PLACEMENT_3D('',#12448,#9868,#9869);
#8477=AXIS2_PLACEMENT_3D('',#12449,#9870,#9871);
#8478=AXIS2_PLACEMENT_3D('',#12452,#9872,#9873);
#8479=AXIS2_PLACEMENT_3D('',#12466,#9876,#9877);
#8480=AXIS2_PLACEMENT_3D('',#12468,#9878,#9879);
#8481=AXIS2_PLACEMENT_3D('',#12470,#9880,#9881);
#8482=AXIS2_PLACEMENT_3D('',#12471,#9882,#9883);
#8483=AXIS2_PLACEMENT_3D('',#12472,#9884,#9885);
#8484=AXIS2_PLACEMENT_3D('',#12477,#9888,#9889);
#8485=AXIS2_PLACEMENT_3D('',#12478,#9890,#9891);
#8486=AXIS2_PLACEMENT_3D('',#12482,#9893,#9894);
#8487=AXIS2_PLACEMENT_3D('',#12493,#9896,#9897);
#8488=AXIS2_PLACEMENT_3D('',#12494,#9898,#9899);
#8489=AXIS2_PLACEMENT_3D('',#12495,#9900,#9901);
#8490=AXIS2_PLACEMENT_3D('',#12499,#9903,#9904);
#8491=AXIS2_PLACEMENT_3D('',#12501,#9906,#9907);
#8492=AXIS2_PLACEMENT_3D('',#12505,#9910,#9911);
#8493=AXIS2_PLACEMENT_3D('',#12510,#9914,#9915);
#8494=AXIS2_PLACEMENT_3D('',#12511,#9916,#9917);
#8495=AXIS2_PLACEMENT_3D('',#12516,#9920,#9921);
#8496=AXIS2_PLACEMENT_3D('',#12517,#9922,#9923);
#8497=AXIS2_PLACEMENT_3D('',#12527,#9929,#9930);
#8498=AXIS2_PLACEMENT_3D('',#12530,#9933,#9934);
#8499=AXIS2_PLACEMENT_3D('',#12533,#9936,#9937);
#8500=AXIS2_PLACEMENT_3D('',#12534,#9938,#9939);
#8501=AXIS2_PLACEMENT_3D('',#12535,#9940,#9941);
#8502=AXIS2_PLACEMENT_3D('',#12546,#9947,#9948);
#8503=AXIS2_PLACEMENT_3D('',#12549,#9950,#9951);
#8504=AXIS2_PLACEMENT_3D('',#12551,#9953,#9954);
#8505=AXIS2_PLACEMENT_3D('',#12553,#9955,#9956);
#8506=AXIS2_PLACEMENT_3D('',#12555,#9958,#9959);
#8507=AXIS2_PLACEMENT_3D('',#12556,#9960,#9961);
#8508=AXIS2_PLACEMENT_3D('',#12560,#9964,#9965);
#8509=AXIS2_PLACEMENT_3D('',#12566,#9969,#9970);
#8510=AXIS2_PLACEMENT_3D('',#12582,#9971,#9972);
#8511=AXIS2_PLACEMENT_3D('',#12583,#9973,#9974);
#8512=AXIS2_PLACEMENT_3D('',#12584,#9975,#9976);
#8513=AXIS2_PLACEMENT_3D('',#12585,#9977,#9978);
#8514=AXIS2_PLACEMENT_3D('',#12589,#9980,#9981);
#8515=AXIS2_PLACEMENT_3D('',#12593,#9983,#9984);
#8516=AXIS2_PLACEMENT_3D('',#12603,#9989,#9990);
#8517=AXIS2_PLACEMENT_3D('',#12606,#9992,#9993);
#8518=AXIS2_PLACEMENT_3D('',#12608,#9994,#9995);
#8519=AXIS2_PLACEMENT_3D('',#12610,#9996,#9997);
#8520=AXIS2_PLACEMENT_3D('',#12611,#9998,#9999);
#8521=AXIS2_PLACEMENT_3D('',#12614,#10000,#10001);
#8522=AXIS2_PLACEMENT_3D('',#12618,#10003,#10004);
#8523=AXIS2_PLACEMENT_3D('',#12620,#10006,#10007);
#8524=AXIS2_PLACEMENT_3D('',#12623,#10010,#10011);
#8525=AXIS2_PLACEMENT_3D('',#12629,#10015,#10016);
#8526=AXIS2_PLACEMENT_3D('',#12631,#10017,#10018);
#8527=AXIS2_PLACEMENT_3D('',#12633,#10019,#10020);
#8528=AXIS2_PLACEMENT_3D('',#12635,#10022,#10023);
#8529=AXIS2_PLACEMENT_3D('',#12638,#10026,#10027);
#8530=AXIS2_PLACEMENT_3D('',#12644,#10031,#10032);
#8531=AXIS2_PLACEMENT_3D('',#12650,#10036,#10037);
#8532=AXIS2_PLACEMENT_3D('',#12652,#10038,#10039);
#8533=AXIS2_PLACEMENT_3D('',#12656,#10041,#10042);
#8534=AXIS2_PLACEMENT_3D('',#12658,#10043,#10044);
#8535=AXIS2_PLACEMENT_3D('',#12666,#10048,#10049);
#8536=AXIS2_PLACEMENT_3D('',#12669,#10051,#10052);
#8537=AXIS2_PLACEMENT_3D('',#12670,#10053,#10054);
#8538=AXIS2_PLACEMENT_3D('',#12673,#10057,#10058);
#8539=AXIS2_PLACEMENT_3D('',#12676,#10061,#10062);
#8540=AXIS2_PLACEMENT_3D('',#12679,#10065,#10066);
#8541=AXIS2_PLACEMENT_3D('',#12682,#10069,#10070);
#8542=AXIS2_PLACEMENT_3D('',#12684,#10072,#10073);
#8543=AXIS2_PLACEMENT_3D('',#12685,#10074,#10075);
#8544=AXIS2_PLACEMENT_3D('',#12686,#10076,#10077);
#8545=AXIS2_PLACEMENT_3D('',#12687,#10078,#10079);
#8546=AXIS2_PLACEMENT_3D('',#12688,#10080,#10081);
#8547=AXIS2_PLACEMENT_3D('',#12689,#10082,#10083);
#8548=AXIS2_PLACEMENT_3D('',#12692,#10085,#10086);
#8549=AXIS2_PLACEMENT_3D('',#12693,#10087,#10088);
#8550=AXIS2_PLACEMENT_3D('',#12694,#10089,#10090);
#8551=AXIS2_PLACEMENT_3D('',#12697,#10092,#10093);
#8552=AXIS2_PLACEMENT_3D('',#12698,#10094,#10095);
#8553=AXIS2_PLACEMENT_3D('',#12699,#10096,#10097);
#8554=AXIS2_PLACEMENT_3D('',#12702,#10099,#10100);
#8555=AXIS2_PLACEMENT_3D('',#12703,#10101,#10102);
#8556=AXIS2_PLACEMENT_3D('',#12704,#10103,#10104);
#8557=AXIS2_PLACEMENT_3D('',#12707,#10106,#10107);
#8558=AXIS2_PLACEMENT_3D('',#12708,#10108,#10109);
#8559=AXIS2_PLACEMENT_3D('',#12709,#10110,#10111);
#8560=AXIS2_PLACEMENT_3D('',#12712,#10112,#10113);
#8561=AXIS2_PLACEMENT_3D('',#12716,#10115,#10116);
#8562=AXIS2_PLACEMENT_3D('',#12718,#10118,#10119);
#8563=AXIS2_PLACEMENT_3D('',#12721,#10120,#10121);
#8564=AXIS2_PLACEMENT_3D('',#12722,#10122,#10123);
#8565=AXIS2_PLACEMENT_3D('',#12723,#10124,#10125);
#8566=AXIS2_PLACEMENT_3D('',#12724,#10126,#10127);
#8567=AXIS2_PLACEMENT_3D('',#12727,#10128,#10129);
#8568=AXIS2_PLACEMENT_3D('',#12741,#10132,#10133);
#8569=AXIS2_PLACEMENT_3D('',#12742,#10134,#10135);
#8570=AXIS2_PLACEMENT_3D('',#12743,#10136,#10137);
#8571=AXIS2_PLACEMENT_3D('',#12744,#10138,#10139);
#8572=AXIS2_PLACEMENT_3D('',#12747,#10140,#10141);
#8573=AXIS2_PLACEMENT_3D('',#12760,#10144,#10145);
#8574=AXIS2_PLACEMENT_3D('',#12761,#10146,#10147);
#8575=AXIS2_PLACEMENT_3D('',#12762,#10148,#10149);
#8576=AXIS2_PLACEMENT_3D('',#12763,#10150,#10151);
#8577=AXIS2_PLACEMENT_3D('',#12765,#10152,#10153);
#8578=AXIS2_PLACEMENT_3D('',#12778,#10155,#10156);
#8579=AXIS2_PLACEMENT_3D('',#12779,#10157,#10158);
#8580=AXIS2_PLACEMENT_3D('',#12780,#10159,#10160);
#8581=AXIS2_PLACEMENT_3D('',#12781,#10161,#10162);
#8582=AXIS2_PLACEMENT_3D('',#12784,#10163,#10164);
#8583=AXIS2_PLACEMENT_3D('',#12797,#10167,#10168);
#8584=AXIS2_PLACEMENT_3D('',#12798,#10169,#10170);
#8585=AXIS2_PLACEMENT_3D('',#12799,#10171,#10172);
#8586=AXIS2_PLACEMENT_3D('',#12800,#10173,#10174);
#8587=AXIS2_PLACEMENT_3D('',#12802,#10175,#10176);
#8588=AXIS2_PLACEMENT_3D('',#12813,#10178,#10179);
#8589=AXIS2_PLACEMENT_3D('',#12814,#10180,#10181);
#8590=AXIS2_PLACEMENT_3D('',#12815,#10182,#10183);
#8591=AXIS2_PLACEMENT_3D('',#12817,#10185,#10186);
#8592=AXIS2_PLACEMENT_3D('',#12819,#10188,#10189);
#8593=AXIS2_PLACEMENT_3D('',#12821,#10191,#10192);
#8594=AXIS2_PLACEMENT_3D('',#12823,#10194,#10195);
#8595=AXIS2_PLACEMENT_3D('',#12825,#10197,#10198);
#8596=AXIS2_PLACEMENT_3D('',#12827,#10200,#10201);
#8597=AXIS2_PLACEMENT_3D('',#12828,#10202,#10203);
#8598=AXIS2_PLACEMENT_3D('',#12829,#10204,#10205);
#8599=AXIS2_PLACEMENT_3D('',#12831,#10207,#10208);
#8600=AXIS2_PLACEMENT_3D('',#12833,#10210,#10211);
#9830=DIRECTION('axis',(0.,0.,1.));
#9831=DIRECTION('refdir',(1.,0.,0.));
#9832=DIRECTION('center_axis',(-1.,0.,0.));
#9833=DIRECTION('ref_axis',(0.,-1.,0.));
#9834=DIRECTION('',(0.,0.,-1.));
#9835=DIRECTION('',(0.,-1.,-3.48381790312471E-17));
#9836=DIRECTION('center_axis',(-1.,0.,0.));
#9837=DIRECTION('ref_axis',(0.,1.,1.66533453693774E-15));
#9838=DIRECTION('',(0.,8.3698837981778E-17,-1.));
#9839=DIRECTION('center_axis',(-1.,0.,0.));
#9840=DIRECTION('ref_axis',(0.,-1.11022302462516E-15,1.));
#9841=DIRECTION('',(0.,1.,0.));
#9842=DIRECTION('center_axis',(-1.,0.,0.));
#9843=DIRECTION('ref_axis',(0.,6.66133814775096E-15,-1.));
#9844=DIRECTION('',(0.,-8.00068553810663E-16,-1.));
#9845=DIRECTION('center_axis',(-1.,0.,0.));
#9846=DIRECTION('ref_axis',(0.,2.2204460492503E-15,1.));
#9847=DIRECTION('',(0.,1.,0.));
#9848=DIRECTION('',(0.,0.,-1.));
#9849=DIRECTION('',(0.,1.,0.));
#9850=DIRECTION('',(0.,-8.00068553810663E-16,-1.));
#9851=DIRECTION('center_axis',(1.,0.,0.));
#9852=DIRECTION('ref_axis',(0.,6.66133814775096E-15,-1.));
#9853=DIRECTION('center_axis',(1.,0.,0.));
#9854=DIRECTION('ref_axis',(0.,1.,0.));
#9855=DIRECTION('',(0.,8.3698837981778E-17,-1.));
#9856=DIRECTION('center_axis',(1.,0.,0.));
#9857=DIRECTION('ref_axis',(0.,1.,0.));
#9858=DIRECTION('center_axis',(-1.,0.,0.));
#9859=DIRECTION('ref_axis',(0.,1.,0.));
#9860=DIRECTION('center_axis',(-1.,0.,0.));
#9861=DIRECTION('ref_axis',(0.,1.,0.));
#9862=DIRECTION('center_axis',(-1.,0.,0.));
#9863=DIRECTION('ref_axis',(0.,0.,-1.));
#9864=DIRECTION('center_axis',(0.,0.,-1.));
#9865=DIRECTION('ref_axis',(-0.258819045102521,-0.965925826289068,0.));
#9866=DIRECTION('center_axis',(1.11022302462516E-15,-1.,0.));
#9867=DIRECTION('ref_axis',(-1.,-1.11022302462516E-15,0.));
#9868=DIRECTION('center_axis',(0.,0.,1.));
#9869=DIRECTION('ref_axis',(-0.258819045102521,-0.965925826289068,0.));
#9870=DIRECTION('center_axis',(-1.,0.,0.));
#9871=DIRECTION('ref_axis',(0.,-0.707106781186547,-0.707106781186548));
#9872=DIRECTION('center_axis',(-1.,0.,0.));
#9873=DIRECTION('ref_axis',(0.,0.,-1.));
#9874=DIRECTION('',(-1.,0.,0.));
#9875=DIRECTION('',(1.,0.,0.));
#9876=DIRECTION('center_axis',(3.33066907387547E-15,1.,-3.69778549322349E-30));
#9877=DIRECTION('ref_axis',(-1.11022302462516E-15,0.,-1.));
#9878=DIRECTION('center_axis',(0.,0.,-1.));
#9879=DIRECTION('ref_axis',(-0.258819045102521,0.965925826289068,0.));
#9880=DIRECTION('center_axis',(-1.,0.,0.));
#9881=DIRECTION('ref_axis',(0.,1.,0.));
#9882=DIRECTION('center_axis',(0.,0.,1.));
#9883=DIRECTION('ref_axis',(-0.258819045102521,0.965925826289068,0.));
#9884=DIRECTION('center_axis',(1.,0.,0.));
#9885=DIRECTION('ref_axis',(0.,0.707106781186547,-0.707106781186548));
#9886=DIRECTION('',(-1.,0.,0.));
#9887=DIRECTION('',(1.,0.,0.));
#9888=DIRECTION('center_axis',(-0.707106781186547,0.707106781186548,-7.85046229341886E-16));
#9889=DIRECTION('ref_axis',(-0.707106781186548,-0.707106781186547,7.85046229341885E-16));
#9890=DIRECTION('center_axis',(0.,-1.,0.));
#9891=DIRECTION('ref_axis',(0.707106781186547,0.,-0.707106781186548));
#9892=DIRECTION('',(0.,-1.,0.));
#9893=DIRECTION('center_axis',(0.,1.,0.));
#9894=DIRECTION('ref_axis',(1.,0.,0.));
#9895=DIRECTION('',(0.,1.,0.));
#9896=DIRECTION('center_axis',(0.,0.,-1.));
#9897=DIRECTION('ref_axis',(0.707106781186548,-0.707106781186548,0.));
#9898=DIRECTION('center_axis',(0.,0.,1.));
#9899=DIRECTION('ref_axis',(0.707106781186547,-0.707106781186547,0.));
#9900=DIRECTION('center_axis',(0.,0.,-1.));
#9901=DIRECTION('ref_axis',(0.,-1.,0.));
#9902=DIRECTION('',(0.,0.,-1.));
#9903=DIRECTION('center_axis',(0.,-3.48381790312471E-17,1.));
#9904=DIRECTION('ref_axis',(0.,-1.,0.));
#9905=DIRECTION('',(0.,0.,-1.));
#9906=DIRECTION('center_axis',(0.,-1.,0.));
#9907=DIRECTION('ref_axis',(-1.,0.,0.));
#9908=DIRECTION('',(0.,0.,-1.));
#9909=DIRECTION('',(1.,0.,0.));
#9910=DIRECTION('center_axis',(0.,0.,-1.));
#9911=DIRECTION('ref_axis',(0.707106781186548,-0.707106781186548,0.));
#9912=DIRECTION('',(0.,0.,1.));
#9913=DIRECTION('',(0.,-1.,-3.48381790312471E-17));
#9914=DIRECTION('center_axis',(0.,-3.48381790312471E-17,1.));
#9915=DIRECTION('ref_axis',(0.707106781186548,-0.707106781186548,0.));
#9916=DIRECTION('center_axis',(1.,0.,0.));
#9917=DIRECTION('ref_axis',(0.,-1.,0.));
#9918=DIRECTION('',(0.,0.,-1.));
#9919=DIRECTION('',(0.,-1.,-3.48381790312471E-17));
#9920=DIRECTION('center_axis',(1.,0.,0.));
#9921=DIRECTION('ref_axis',(0.,-1.,0.));
#9922=DIRECTION('center_axis',(0.,-1.,0.));
#9923=DIRECTION('ref_axis',(1.,0.,0.));
#9924=DIRECTION('',(0.,0.,-1.));
#9925=DIRECTION('',(1.,0.,0.));
#9926=DIRECTION('',(0.,0.,1.));
#9927=DIRECTION('',(-1.,0.,0.));
#9928=DIRECTION('',(0.,0.,1.));
#9929=DIRECTION('center_axis',(0.,1.,0.));
#9930=DIRECTION('ref_axis',(-0.707106781186548,0.,-0.707106781186548));
#9931=DIRECTION('',(0.,1.,0.));
#9932=DIRECTION('',(0.,-1.,0.));
#9933=DIRECTION('center_axis',(0.,0.,-1.));
#9934=DIRECTION('ref_axis',(-1.,1.66533453693773E-15,0.));
#9935=DIRECTION('',(0.,0.,-1.));
#9936=DIRECTION('center_axis',(0.,-3.48381790312471E-17,1.));
#9937=DIRECTION('ref_axis',(-1.,1.66533453693773E-15,0.));
#9938=DIRECTION('center_axis',(0.,0.,-1.));
#9939=DIRECTION('ref_axis',(1.,0.,0.));
#9940=DIRECTION('center_axis',(0.,3.48381790312471E-17,-1.));
#9941=DIRECTION('ref_axis',(0.,-1.,-3.48381790312471E-17));
#9942=DIRECTION('',(0.,-1.,-3.48381790312471E-17));
#9943=DIRECTION('',(-1.,0.,0.));
#9944=DIRECTION('',(0.,-1.,-3.48381790312471E-17));
#9945=DIRECTION('',(-1.,0.,0.));
#9946=DIRECTION('',(-1.,0.,0.));
#9947=DIRECTION('center_axis',(0.,-3.48381790312471E-17,1.));
#9948=DIRECTION('ref_axis',(-1.,0.,0.));
#9949=DIRECTION('',(0.,-1.,-3.48381790312471E-17));
#9950=DIRECTION('center_axis',(0.,-3.48381790312471E-17,1.));
#9951=DIRECTION('ref_axis',(2.22044604925031E-15,-1.,0.));
#9952=DIRECTION('',(0.,-1.,-3.48381790312471E-17));
#9953=DIRECTION('center_axis',(1.,0.,0.));
#9954=DIRECTION('ref_axis',(0.,-1.,0.));
#9955=DIRECTION('center_axis',(1.,0.,0.));
#9956=DIRECTION('ref_axis',(0.,-1.,0.));
#9957=DIRECTION('',(1.,0.,0.));
#9958=DIRECTION('center_axis',(-1.,0.,0.));
#9959=DIRECTION('ref_axis',(0.,1.,0.));
#9960=DIRECTION('center_axis',(0.,1.,0.));
#9961=DIRECTION('ref_axis',(-1.,0.,0.));
#9962=DIRECTION('',(1.,0.,0.));
#9963=DIRECTION('',(0.,0.,1.));
#9964=DIRECTION('center_axis',(-1.,0.,0.));
#9965=DIRECTION('ref_axis',(0.,-1.,0.));
#9966=DIRECTION('',(0.,0.,1.));
#9967=DIRECTION('',(0.,1.,3.48381790312471E-17));
#9968=DIRECTION('',(0.,0.,1.));
#9969=DIRECTION('center_axis',(0.,0.,1.));
#9970=DIRECTION('ref_axis',(-1.,0.,0.));
#9971=DIRECTION('center_axis',(0.,3.48381790312471E-17,-1.));
#9972=DIRECTION('ref_axis',(-1.,0.,0.));
#9973=DIRECTION('center_axis',(0.,0.,1.));
#9974=DIRECTION('ref_axis',(2.22044604925031E-15,-1.,0.));
#9975=DIRECTION('center_axis',(0.,3.48381790312471E-17,-1.));
#9976=DIRECTION('ref_axis',(2.22044604925031E-15,-1.,0.));
#9977=DIRECTION('center_axis',(-1.,0.,0.));
#9978=DIRECTION('ref_axis',(0.,-1.,0.));
#9979=DIRECTION('',(0.,-1.,-3.48381790312471E-17));
#9980=DIRECTION('center_axis',(1.,0.,0.));
#9981=DIRECTION('ref_axis',(0.,1.,0.));
#9982=DIRECTION('',(0.,-3.17503269079253E-17,1.));
#9983=DIRECTION('center_axis',(1.,0.,0.));
#9984=DIRECTION('ref_axis',(0.,1.,0.));
#9985=DIRECTION('',(0.,-3.17503269079253E-17,1.));
#9986=DIRECTION('',(0.,1.,0.));
#9987=DIRECTION('',(0.,0.,1.));
#9988=DIRECTION('',(0.,1.,0.));
#9989=DIRECTION('center_axis',(-1.,0.,0.));
#9990=DIRECTION('ref_axis',(0.,-1.,0.));
#9991=DIRECTION('',(0.,-3.17503269079253E-17,1.));
#9992=DIRECTION('center_axis',(-1.,0.,0.));
#9993=DIRECTION('ref_axis',(0.,2.22044604925032E-15,-1.));
#9994=DIRECTION('center_axis',(-1.,0.,0.));
#9995=DIRECTION('ref_axis',(0.,1.,0.));
#9996=DIRECTION('center_axis',(-1.,0.,0.));
#9997=DIRECTION('ref_axis',(0.,1.,0.));
#9998=DIRECTION('center_axis',(0.,0.,-1.));
#9999=DIRECTION('ref_axis',(-1.,1.11022302462516E-15,0.));
#10000=DIRECTION('center_axis',(0.,0.,1.));
#10001=DIRECTION('ref_axis',(-1.,1.11022302462516E-15,0.));
#10002=DIRECTION('',(0.,0.,-1.));
#10003=DIRECTION('center_axis',(0.,0.,-1.));
#10004=DIRECTION('ref_axis',(-1.,1.11022302462516E-15,0.));
#10005=DIRECTION('',(0.,0.,-1.));
#10006=DIRECTION('center_axis',(-1.11022302462516E-16,-1.,0.));
#10007=DIRECTION('ref_axis',(-1.,1.11022302462516E-16,0.));
#10008=DIRECTION('',(1.,-1.11022302462516E-16,0.));
#10009=DIRECTION('',(-1.,1.11022302462516E-16,0.));
#10010=DIRECTION('center_axis',(0.,1.,0.));
#10011=DIRECTION('ref_axis',(1.,0.,0.));
#10012=DIRECTION('',(-1.,0.,0.));
#10013=DIRECTION('',(1.,0.,0.));
#10014=DIRECTION('',(0.,0.,-1.));
#10015=DIRECTION('center_axis',(0.,0.,-1.));
#10016=DIRECTION('ref_axis',(1.11022302462516E-15,1.,0.));
#10017=DIRECTION('center_axis',(0.,0.,1.));
#10018=DIRECTION('ref_axis',(1.11022302462516E-15,1.,0.));
#10019=DIRECTION('center_axis',(0.,0.,-1.));
#10020=DIRECTION('ref_axis',(1.11022302462516E-15,1.,0.));
#10021=DIRECTION('',(0.,0.,-1.));
#10022=DIRECTION('center_axis',(-1.,0.,0.));
#10023=DIRECTION('ref_axis',(0.,1.,0.));
#10024=DIRECTION('',(0.,-1.,0.));
#10025=DIRECTION('',(0.,1.,0.));
#10026=DIRECTION('center_axis',(0.,0.,1.));
#10027=DIRECTION('ref_axis',(0.,1.,0.));
#10028=DIRECTION('',(-1.,0.,0.));
#10029=DIRECTION('',(0.,1.,0.));
#10030=DIRECTION('',(-1.,0.,0.));
#10031=DIRECTION('center_axis',(0.,3.48381790312471E-17,-1.));
#10032=DIRECTION('ref_axis',(0.,-1.,-3.48381790312471E-17));
#10033=DIRECTION('',(-1.,0.,0.));
#10034=DIRECTION('',(0.,-1.,-3.48381790312471E-17));
#10035=DIRECTION('',(1.,0.,0.));
#10036=DIRECTION('center_axis',(-1.,0.,0.));
#10037=DIRECTION('ref_axis',(0.,-1.,0.));
#10038=DIRECTION('center_axis',(-1.,0.,0.));
#10039=DIRECTION('ref_axis',(0.,1.,0.));
#10040=DIRECTION('',(0.,-8.3698837981778E-17,1.));
#10041=DIRECTION('center_axis',(-1.,0.,0.));
#10042=DIRECTION('ref_axis',(0.,1.,0.));
#10043=DIRECTION('center_axis',(-1.,0.,0.));
#10044=DIRECTION('ref_axis',(0.,6.66133814775096E-15,-1.));
#10045=DIRECTION('',(0.,8.00068553810663E-16,1.));
#10046=DIRECTION('',(0.,1.,0.));
#10047=DIRECTION('',(0.,-3.17503269079253E-17,1.));
#10048=DIRECTION('center_axis',(-1.,0.,0.));
#10049=DIRECTION('ref_axis',(0.,1.,0.));
#10050=DIRECTION('',(0.,-3.17503269079253E-17,1.));
#10051=DIRECTION('center_axis',(-1.,0.,0.));
#10052=DIRECTION('ref_axis',(0.,1.,0.));
#10053=DIRECTION('center_axis',(0.,1.,8.3698837981778E-17));
#10054=DIRECTION('ref_axis',(0.,8.3698837981778E-17,-1.));
#10055=DIRECTION('',(1.,0.,0.));
#10056=DIRECTION('',(-1.,0.,0.));
#10057=DIRECTION('center_axis',(0.,-1.,-3.17503269079253E-17));
#10058=DIRECTION('ref_axis',(0.,-3.17503269079253E-17,1.));
#10059=DIRECTION('',(-1.,0.,0.));
#10060=DIRECTION('',(1.,0.,0.));
#10061=DIRECTION('center_axis',(0.,-1.,-3.17503269079253E-17));
#10062=DIRECTION('ref_axis',(0.,-3.17503269079253E-17,1.));
#10063=DIRECTION('',(1.,0.,0.));
#10064=DIRECTION('',(-1.,0.,0.));
#10065=DIRECTION('center_axis',(-1.,0.,0.));
#10066=DIRECTION('ref_axis',(0.,6.66133814775096E-15,-1.));
#10067=DIRECTION('',(1.,0.,0.));
#10068=DIRECTION('',(-1.,0.,0.));
#10069=DIRECTION('center_axis',(0.,0.,1.));
#10070=DIRECTION('ref_axis',(0.,1.,0.));
#10071=DIRECTION('',(1.,0.,0.));
#10072=DIRECTION('center_axis',(-1.,0.,0.));
#10073=DIRECTION('ref_axis',(0.,-0.715401949147516,-0.69871313938979));
#10074=DIRECTION('center_axis',(-1.,0.,0.));
#10075=DIRECTION('ref_axis',(0.,1.,0.));
#10076=DIRECTION('center_axis',(-1.,0.,0.));
#10077=DIRECTION('ref_axis',(0.,1.,0.));
#10078=DIRECTION('center_axis',(-1.,0.,0.));
#10079=DIRECTION('ref_axis',(0.,-0.728392179415956,0.685160443228937));
#10080=DIRECTION('center_axis',(0.,1.,-8.00068553810663E-16));
#10081=DIRECTION('ref_axis',(0.,-8.00068553810663E-16,-1.));
#10082=DIRECTION('center_axis',(-1.,0.,0.));
#10083=DIRECTION('ref_axis',(0.,1.,0.));
#10084=DIRECTION('',(-1.,0.,0.));
#10085=DIRECTION('center_axis',(-1.,0.,0.));
#10086=DIRECTION('ref_axis',(0.,1.,0.));
#10087=DIRECTION('center_axis',(1.,0.,0.));
#10088=DIRECTION('ref_axis',(0.,1.,0.));
#10089=DIRECTION('center_axis',(-1.,0.,0.));
#10090=DIRECTION('ref_axis',(0.,1.,0.));
#10091=DIRECTION('',(-1.,0.,0.));
#10092=DIRECTION('center_axis',(-1.,0.,0.));
#10093=DIRECTION('ref_axis',(0.,1.,0.));
#10094=DIRECTION('center_axis',(1.,0.,0.));
#10095=DIRECTION('ref_axis',(0.,1.,0.));
#10096=DIRECTION('center_axis',(-1.,0.,0.));
#10097=DIRECTION('ref_axis',(0.,1.,0.));
#10098=DIRECTION('',(-1.,0.,0.));
#10099=DIRECTION('center_axis',(-1.,0.,0.));
#10100=DIRECTION('ref_axis',(0.,1.,0.));
#10101=DIRECTION('center_axis',(1.,0.,0.));
#10102=DIRECTION('ref_axis',(0.,1.,0.));
#10103=DIRECTION('center_axis',(-1.,0.,0.));
#10104=DIRECTION('ref_axis',(0.,1.,0.));
#10105=DIRECTION('',(-1.,0.,0.));
#10106=DIRECTION('center_axis',(-1.,0.,0.));
#10107=DIRECTION('ref_axis',(0.,1.,0.));
#10108=DIRECTION('center_axis',(1.,0.,0.));
#10109=DIRECTION('ref_axis',(0.,1.,0.));
#10110=DIRECTION('center_axis',(0.,-8.00068553810663E-16,-1.));
#10111=DIRECTION('ref_axis',(-0.707106781186546,0.707106781186549,0.));
#10112=DIRECTION('center_axis',(0.,0.,-1.));
#10113=DIRECTION('ref_axis',(-1.,0.,0.));
#10114=DIRECTION('',(0.,-8.00068553810663E-16,-1.));
#10115=DIRECTION('center_axis',(0.,0.,1.));
#10116=DIRECTION('ref_axis',(0.,1.,0.));
#10117=DIRECTION('',(0.,8.00068553810663E-16,1.));
#10118=DIRECTION('center_axis',(1.,0.,0.));
#10119=DIRECTION('ref_axis',(0.,0.,-1.));
#10120=DIRECTION('center_axis',(0.,-1.,-6.66133814775096E-15));
#10121=DIRECTION('ref_axis',(0.,-6.66133814775096E-15,1.));
#10122=DIRECTION('center_axis',(-1.,0.,0.));
#10123=DIRECTION('ref_axis',(0.,-0.707106781186542,-0.707106781186553));
#10124=DIRECTION('center_axis',(1.,0.,0.));
#10125=DIRECTION('ref_axis',(0.,-0.707106781186542,-0.707106781186553));
#10126=DIRECTION('center_axis',(0.,1.,0.));
#10127=DIRECTION('ref_axis',(-0.707106781186549,0.,0.707106781186546));
#10128=DIRECTION('center_axis',(0.,-1.,0.));
#10129=DIRECTION('ref_axis',(0.,0.,1.));
#10130=DIRECTION('',(0.,-1.,0.));
#10131=DIRECTION('',(0.,1.,0.));
#10132=DIRECTION('center_axis',(0.,8.88178419700124E-15,1.));
#10133=DIRECTION('ref_axis',(0.,1.,-8.88178419700124E-15));
#10134=DIRECTION('center_axis',(1.,0.,0.));
#10135=DIRECTION('ref_axis',(0.,0.707106781186551,0.707106781186544));
#10136=DIRECTION('center_axis',(-1.,0.,0.));
#10137=DIRECTION('ref_axis',(0.,0.707106781186551,0.707106781186544));
#10138=DIRECTION('center_axis',(0.,8.3698837981778E-17,-1.));
#10139=DIRECTION('ref_axis',(-0.707106781186546,0.707106781186549,0.));
#10140=DIRECTION('center_axis',(0.,0.,1.));
#10141=DIRECTION('ref_axis',(0.,1.,0.));
#10142=DIRECTION('',(0.,-8.3698837981778E-17,1.));
#10143=DIRECTION('',(0.,8.3698837981778E-17,-1.));
#10144=DIRECTION('center_axis',(0.,1.,-2.22044604925031E-15));
#10145=DIRECTION('ref_axis',(0.,-2.22044604925031E-15,-1.));
#10146=DIRECTION('center_axis',(1.,0.,0.));
#10147=DIRECTION('ref_axis',(0.,0.707106781186549,-0.707106781186547));
#10148=DIRECTION('center_axis',(-1.,0.,0.));
#10149=DIRECTION('ref_axis',(0.,0.707106781186548,-0.707106781186547));
#10150=DIRECTION('center_axis',(0.,-1.,-3.48381790312471E-17));
#10151=DIRECTION('ref_axis',(-0.707106781186548,0.,-0.707106781186547));
#10152=DIRECTION('center_axis',(0.,1.,2.22044604925031E-15));
#10153=DIRECTION('ref_axis',(0.,2.22044604925031E-15,-1.));
#10154=DIRECTION('',(0.,1.,3.48381790312471E-17));
#10155=DIRECTION('center_axis',(0.,-8.32667268468869E-16,-1.));
#10156=DIRECTION('ref_axis',(0.,-1.,8.32667268468868E-16));
#10157=DIRECTION('center_axis',(1.,0.,0.));
#10158=DIRECTION('ref_axis',(0.,-0.707106781186547,-0.707106781186548));
#10159=DIRECTION('center_axis',(-1.,0.,0.));
#10160=DIRECTION('ref_axis',(0.,-0.707106781186547,-0.707106781186548));
#10161=DIRECTION('center_axis',(0.,-3.17503269079253E-17,1.));
#10162=DIRECTION('ref_axis',(-0.707106781186549,-0.707106781186546,0.));
#10163=DIRECTION('center_axis',(0.,0.,-1.));
#10164=DIRECTION('ref_axis',(0.,-1.,0.));
#10165=DIRECTION('',(0.,3.17503269079253E-17,-1.));
#10166=DIRECTION('',(0.,-3.17503269079253E-17,1.));
#10167=DIRECTION('center_axis',(0.,-1.,0.));
#10168=DIRECTION('ref_axis',(0.,0.,1.));
#10169=DIRECTION('center_axis',(1.,0.,0.));
#10170=DIRECTION('ref_axis',(0.,-0.707106781186547,0.707106781186548));
#10171=DIRECTION('center_axis',(-1.,0.,0.));
#10172=DIRECTION('ref_axis',(0.,-0.707106781186547,0.707106781186548));
#10173=DIRECTION('center_axis',(0.,1.,0.));
#10174=DIRECTION('ref_axis',(-0.707106781186549,0.,0.707106781186546));
#10175=DIRECTION('center_axis',(0.,-1.,0.));
#10176=DIRECTION('ref_axis',(0.,0.,1.));
#10177=DIRECTION('',(0.,-1.,0.));
#10178=DIRECTION('center_axis',(1.,0.,0.));
#10179=DIRECTION('ref_axis',(0.,0.707106781186545,0.70710678118655));
#10180=DIRECTION('center_axis',(-1.,0.,0.));
#10181=DIRECTION('ref_axis',(0.,0.707106781186545,0.70710678118655));
#10182=DIRECTION('center_axis',(-1.,0.,0.));
#10183=DIRECTION('ref_axis',(0.,1.,1.66533453693774E-15));
#10184=DIRECTION('',(-1.,0.,0.));
#10185=DIRECTION('center_axis',(0.,1.,8.3698837981778E-17));
#10186=DIRECTION('ref_axis',(0.,8.3698837981778E-17,-1.));
#10187=DIRECTION('',(-1.,0.,0.));
#10188=DIRECTION('center_axis',(-1.,0.,0.));
#10189=DIRECTION('ref_axis',(0.,-1.11022302462516E-15,1.));
#10190=DIRECTION('',(-1.,0.,0.));
#10191=DIRECTION('center_axis',(0.,0.,1.));
#10192=DIRECTION('ref_axis',(0.,1.,0.));
#10193=DIRECTION('',(-1.,0.,0.));
#10194=DIRECTION('center_axis',(-1.,0.,0.));
#10195=DIRECTION('ref_axis',(0.,6.66133814775096E-15,-1.));
#10196=DIRECTION('',(-1.,0.,0.));
#10197=DIRECTION('center_axis',(0.,1.,-8.00068553810663E-16));
#10198=DIRECTION('ref_axis',(0.,-8.00068553810663E-16,-1.));
#10199=DIRECTION('',(-1.,0.,0.));
#10200=DIRECTION('center_axis',(-1.,0.,0.));
#10201=DIRECTION('ref_axis',(0.,-1.,0.));
#10202=DIRECTION('center_axis',(-1.,0.,0.));
#10203=DIRECTION('ref_axis',(0.,2.2204460492503E-15,1.));
#10204=DIRECTION('center_axis',(-1.,0.,0.));
#10205=DIRECTION('ref_axis',(0.,-1.,0.));
#10206=DIRECTION('',(-1.,0.,0.));
#10207=DIRECTION('center_axis',(0.,-1.,-3.17503269079253E-17));
#10208=DIRECTION('ref_axis',(0.,-3.17503269079253E-17,1.));
#10209=DIRECTION('',(-1.,0.,0.));
#10210=DIRECTION('center_axis',(-1.,0.,0.));
#10211=DIRECTION('ref_axis',(0.,2.22044604925032E-15,-1.));
#12392=CARTESIAN_POINT('',(0.,0.,0.));
#12393=CARTESIAN_POINT('Origin',(-0.499999999999999,9.50222608824143,11.9189153104842));
#12394=CARTESIAN_POINT('',(-0.499999999999999,22.2688065021356,-20.2341199955735));
#12395=CARTESIAN_POINT('',(-0.5,22.2688065021356,-25.0483789742253));
#12396=CARTESIAN_POINT('',(-0.499999999999999,22.2688065021356,-6.56473183187052));
#12397=CARTESIAN_POINT('',(-0.499999999999999,25.4362251590507,-25.0483789742253));
#12398=CARTESIAN_POINT('',(-0.499999999999999,25.4362251590507,-25.0483789742253));
#12399=CARTESIAN_POINT('',(-0.499999999999999,27.4362251590507,-23.0483789742253));
#12400=CARTESIAN_POINT('Origin',(-0.499999999999999,25.4362251590507,-23.0483789742253));
#12401=CARTESIAN_POINT('',(-0.499999999999999,27.4362251590507,30.0096109045284));
#12402=CARTESIAN_POINT('',(-0.499999999999999,27.4362251590507,30.0096109045284));
#12403=CARTESIAN_POINT('',(-0.499999999999999,25.4362251590507,32.0096109045284));
#12404=CARTESIAN_POINT('Origin',(-0.499999999999999,25.4362251590507,30.0096109045284));
#12405=CARTESIAN_POINT('',(-0.499999999999999,22.2953189477036,32.0096109045284));
#12406=CARTESIAN_POINT('',(-0.499999999999999,22.2953189477036,32.0096109045284));
#12407=CARTESIAN_POINT('',(-0.499999999999999,21.2953189477036,33.0096109045284));
#12408=CARTESIAN_POINT('Origin',(-0.499999999999999,22.2953189477035,33.0096109045284));
#12409=CARTESIAN_POINT('',(-0.499999999999999,21.2953189477036,46.8862095951938));
#12410=CARTESIAN_POINT('',(-0.499999999999999,21.2953189477036,46.8862095951938));
#12411=CARTESIAN_POINT('',(-0.499999999999999,19.2953189477036,48.8862095951938));
#12412=CARTESIAN_POINT('Origin',(-0.499999999999999,19.2953189477036,46.8862095951938));
#12413=CARTESIAN_POINT('',(-0.499999999999999,18.4317729825679,48.8862095951938));
#12414=CARTESIAN_POINT('',(-0.499999999999999,-6.43177298256785,48.8862095951938));
#12415=CARTESIAN_POINT('',(-0.499999999999999,18.4317729825679,46.8862095951938));
#12416=CARTESIAN_POINT('',(-0.499999999999999,18.4317729825679,30.402562452839));
#12417=CARTESIAN_POINT('',(-0.499999999999999,19.2953189477036,46.8862095951938));
#12418=CARTESIAN_POINT('',(-0.499999999999999,1.53522655283679,46.8862095951938));
#12419=CARTESIAN_POINT('',(-0.499999999999999,19.2953189477036,33.0096109045284));
#12420=CARTESIAN_POINT('',(-0.499999999999999,19.2953189477035,29.402562452839));
#12421=CARTESIAN_POINT('',(-0.499999999999999,21.4945386978003,30.1184604429708));
#12422=CARTESIAN_POINT('Origin',(-0.499999999999999,22.2953189477035,33.0096109045284));
#12423=CARTESIAN_POINT('',(-0.499999999999999,25.4362251590507,26.0826265387027));
#12424=CARTESIAN_POINT('Origin',(-0.499999999999999,24.9477990585308,29.5483789742253));
#12425=CARTESIAN_POINT('',(-0.499999999999999,25.4362251590507,-18.9365770263474));
#12426=CARTESIAN_POINT('',(-0.499999999999999,25.4362251590507,20.9642631075063));
#12427=CARTESIAN_POINT('Origin',(-0.499999999999999,25.0098518119976,-22.4105093470644));
#12428=CARTESIAN_POINT('',(-0.499999999999999,23.4477990585308,29.5483789742253));
#12429=CARTESIAN_POINT('Origin',(-0.499999999999999,24.9477990585308,29.5483789742253));
#12430=CARTESIAN_POINT('',(-0.499999999999999,23.5098518119976,-22.4105093470644));
#12431=CARTESIAN_POINT('Origin',(-0.499999999999999,25.0098518119976,-22.4105093470644));
#12432=CARTESIAN_POINT('Ctrl Pts',(-13.112465101899,-4.10380624392837,-40.0483789742253));
#12433=CARTESIAN_POINT('Ctrl Pts',(-15.112465101899,-4.10380624392837,-40.0483789742253));
#12434=CARTESIAN_POINT('Ctrl Pts',(-15.112465101899,-2.10380624392837,-40.0483789742253));
#12435=CARTESIAN_POINT('Ctrl Pts',(-13.112465101899,-4.10380624392837,-41.0483789742253));
#12436=CARTESIAN_POINT('Ctrl Pts',(-15.112465101899,-4.10380624392837,-41.0483789742253));
#12437=CARTESIAN_POINT('Ctrl Pts',(-15.112465101899,-2.10380624392837,-41.0483789742253));
#12438=CARTESIAN_POINT('Ctrl Pts',(-13.112465101899,-3.10380624392837,-41.0483789742253));
#12439=CARTESIAN_POINT('Ctrl Pts',(-14.112465101899,-3.10380624392837,-41.0483789742253));
#12440=CARTESIAN_POINT('Ctrl Pts',(-14.112465101899,-2.10380624392837,-41.0483789742253));
#12441=CARTESIAN_POINT('',(-13.112465101899,-3.10380624392837,-41.0483789742253));
#12442=CARTESIAN_POINT('',(-13.112465101899,-4.10380624392837,-40.0483789742253));
#12443=CARTESIAN_POINT('Origin',(-13.112465101899,-3.10380624392837,-40.0483789742253));
#12444=CARTESIAN_POINT('',(-15.112465101899,-2.10380624392837,-40.0483789742253));
#12445=CARTESIAN_POINT('Origin',(-13.112465101899,-2.10380624392837,-40.0483789742253));
#12446=CARTESIAN_POINT('',(-14.112465101899,-2.10380624392837,-41.0483789742253));
#12447=CARTESIAN_POINT('Origin',(-14.112465101899,-2.10380624392837,-40.0483789742253));
#12448=CARTESIAN_POINT('Origin',(-13.112465101899,-2.10380624392837,-41.0483789742253));
#12449=CARTESIAN_POINT('Origin',(-5.56259599847326,-3.10380624392837,-40.0483789742253));
#12450=CARTESIAN_POINT('',(-2.49997296399801,-3.10380624392837,-41.0483789742253));
#12451=CARTESIAN_POINT('',(-2.49997296399801,-4.10380624392837,-40.0483789742253));
#12452=CARTESIAN_POINT('Origin',(-2.49997296399801,-3.10380624392837,-40.0483789742253));
#12453=CARTESIAN_POINT('',(-5.56259599847326,-4.10380624392837,-40.0483789742253));
#12454=CARTESIAN_POINT('',(-5.56259599847326,-3.10380624392837,-41.0483789742253));
#12455=CARTESIAN_POINT('Ctrl Pts',(-15.112465101899,14.8031072225088,-40.0483789742253));
#12456=CARTESIAN_POINT('Ctrl Pts',(-15.112465101899,16.8031072225088,-40.0483789742253));
#12457=CARTESIAN_POINT('Ctrl Pts',(-13.112465101899,16.8031072225088,-40.0483789742253));
#12458=CARTESIAN_POINT('Ctrl Pts',(-15.112465101899,14.8031072225088,-41.0483789742253));
#12459=CARTESIAN_POINT('Ctrl Pts',(-15.112465101899,16.8031072225088,-41.0483789742253));
#12460=CARTESIAN_POINT('Ctrl Pts',(-13.112465101899,16.8031072225088,-41.0483789742253));
#12461=CARTESIAN_POINT('Ctrl Pts',(-14.112465101899,14.8031072225088,-41.0483789742253));
#12462=CARTESIAN_POINT('Ctrl Pts',(-14.112465101899,15.8031072225088,-41.0483789742253));
#12463=CARTESIAN_POINT('Ctrl Pts',(-13.112465101899,15.8031072225088,-41.0483789742253));
#12464=CARTESIAN_POINT('',(-14.112465101899,14.8031072225088,-41.0483789742253));
#12465=CARTESIAN_POINT('',(-15.112465101899,14.8031072225088,-40.0483789742253));
#12466=CARTESIAN_POINT('Origin',(-14.112465101899,14.8031072225088,-40.0483789742253));
#12467=CARTESIAN_POINT('',(-13.112465101899,16.8031072225088,-40.0483789742253));
#12468=CARTESIAN_POINT('Origin',(-13.112465101899,14.8031072225088,-40.0483789742253));
#12469=CARTESIAN_POINT('',(-13.112465101899,15.8031072225088,-41.0483789742253));
#12470=CARTESIAN_POINT('Origin',(-13.112465101899,15.8031072225088,-40.0483789742253));
#12471=CARTESIAN_POINT('Origin',(-13.112465101899,14.8031072225088,-41.0483789742253));
#12472=CARTESIAN_POINT('Origin',(-11.4097522506131,15.8031073387245,-40.0483789742253));
#12473=CARTESIAN_POINT('',(-1.49997296399801,15.8031073387245,-41.0483789742253));
#12474=CARTESIAN_POINT('',(-11.4097522506131,15.8031073387245,-41.0483789742253));
#12475=CARTESIAN_POINT('',(-0.499972963998009,16.8031073387245,-40.0483789742253));
#12476=CARTESIAN_POINT('',(-11.4097522506131,16.8031073387245,-40.0483789742253));
#12477=CARTESIAN_POINT('Origin',(-1.49997296399801,15.8031073387245,-40.0483789742253));
#12478=CARTESIAN_POINT('Origin',(-1.49997296399801,10.5763788558995,-40.0483789742253));
#12479=CARTESIAN_POINT('',(-0.499972963998009,-2.10380624392837,-40.0483789742253));
#12480=CARTESIAN_POINT('',(-0.499972963998009,10.5763788558995,-40.0483789742253));
#12481=CARTESIAN_POINT('',(-1.49997296399801,-2.10380624392837,-41.0483789742253));
#12482=CARTESIAN_POINT('Origin',(-1.49997296399801,-2.10380624392837,-40.0483789742253));
#12483=CARTESIAN_POINT('',(-1.49997296399801,10.5763788558995,-41.0483789742253));
#12484=CARTESIAN_POINT('Ctrl Pts',(-2.49997296399801,-3.10380624392837,
-41.0483789742253));
#12485=CARTESIAN_POINT('Ctrl Pts',(-1.49997296399801,-3.10380624392837,
-41.0483789742253));
#12486=CARTESIAN_POINT('Ctrl Pts',(-1.49997296399801,-2.10380624392837,
-41.0483789742253));
#12487=CARTESIAN_POINT('Ctrl Pts',(-2.49997296399801,-4.10380624392837,
-41.0483789742253));
#12488=CARTESIAN_POINT('Ctrl Pts',(-0.499972963998009,-4.10380624392837,
-41.0483789742253));
#12489=CARTESIAN_POINT('Ctrl Pts',(-0.499972963998009,-2.10380624392837,
-41.0483789742253));
#12490=CARTESIAN_POINT('Ctrl Pts',(-2.49997296399801,-4.10380624392837,
-40.0483789742253));
#12491=CARTESIAN_POINT('Ctrl Pts',(-0.499972963998009,-4.10380624392837,
-40.0483789742253));
#12492=CARTESIAN_POINT('Ctrl Pts',(-0.499972963998009,-2.10380624392837,
-40.0483789742253));
#12493=CARTESIAN_POINT('Origin',(-2.49997296399801,-2.10380624392837,-40.0483789742253));
#12494=CARTESIAN_POINT('Origin',(-2.49997296399801,-2.10380624392837,-41.0483789742253));
#12495=CARTESIAN_POINT('Origin',(-13.112465101899,-2.10380624392837,-25.0483789742253));
#12496=CARTESIAN_POINT('',(-13.112465101899,-4.10380624392837,-25.0483789742253));
#12497=CARTESIAN_POINT('',(-13.112465101899,-4.10380624392837,-25.0483789742253));
#12498=CARTESIAN_POINT('',(-15.112465101899,-2.10380624392837,-25.0483789742253));
#12499=CARTESIAN_POINT('Origin',(-13.112465101899,-2.10380624392837,-25.0483789742253));
#12500=CARTESIAN_POINT('',(-15.112465101899,-2.10380624392837,-25.0483789742253));
#12501=CARTESIAN_POINT('Origin',(-3.04597296399801,-4.10380624392837,-25.0483789742253));
#12502=CARTESIAN_POINT('',(-2.49997296399801,-4.10380624392837,-25.0483789742253));
#12503=CARTESIAN_POINT('',(-2.49997296399801,-4.10380624392837,-25.0483789742253));
#12504=CARTESIAN_POINT('',(-1.772986481999,-4.10380624392837,-25.0483789742253));
#12505=CARTESIAN_POINT('Origin',(-2.49997296399801,-2.10380624392837,-25.0483789742253));
#12506=CARTESIAN_POINT('',(-0.499999999999999,-2.10380624392837,-25.0483789742253));
#12507=CARTESIAN_POINT('',(-0.499972963998009,-2.10380624392837,-25.0483789742253));
#12508=CARTESIAN_POINT('',(-0.499999999999999,-2.11420543990764,-25.0483789742253));
#12509=CARTESIAN_POINT('',(-0.499999999999999,25.4362251590507,-25.0483789742253));
#12510=CARTESIAN_POINT('Origin',(-2.49997296399801,-2.10380624392837,-25.0483789742253));
#12511=CARTESIAN_POINT('Origin',(-0.499972963998009,14.8031072225088,-25.0483789742253));
#12512=CARTESIAN_POINT('',(-0.499999999999999,16.8031073387245,-25.0483789742253));
#12513=CARTESIAN_POINT('',(-0.499972963998009,16.8031073387245,-25.0483789742253));
#12514=CARTESIAN_POINT('',(-0.499999999999999,25.4362251590507,-25.0483789742253));
#12515=CARTESIAN_POINT('',(-0.499972963998008,10.4317729825678,-32.9865355928432));
#12516=CARTESIAN_POINT('Origin',(-0.499972963998008,6.43177298256785,-32.9865355928432));
#12517=CARTESIAN_POINT('Origin',(-14.7402854682776,16.8031073387245,-25.0483789742253));
#12518=CARTESIAN_POINT('',(-13.112465101899,16.8031072225088,-25.0483789742253));
#12519=CARTESIAN_POINT('',(-13.112465101899,16.8031072225088,-25.0483789742253));
#12520=CARTESIAN_POINT('',(-14.7402854682776,16.8031073387245,-25.0483789742253));
#12521=CARTESIAN_POINT('',(-7.62014273413882,16.8031073387245,-25.0483789742253));
#12522=CARTESIAN_POINT('',(-14.7402854682776,16.8031073387245,-23.0483789742253));
#12523=CARTESIAN_POINT('',(-14.7402854682776,16.8031073387245,-25.0483789742253));
#12524=CARTESIAN_POINT('',(-0.499999999999999,16.8031073387245,-23.0483789742253));
#12525=CARTESIAN_POINT('',(-7.62014273413882,16.8031073387245,-23.0483789742253));
#12526=CARTESIAN_POINT('',(-0.499999999999999,16.8031073387245,-6.56473183187052));
#12527=CARTESIAN_POINT('Origin',(-14.112465101899,2.12292212268092,-40.0483789742253));
#12528=CARTESIAN_POINT('',(-15.112465101899,2.12292212268092,-40.0483789742253));
#12529=CARTESIAN_POINT('',(-14.112465101899,2.12292212268092,-41.0483789742253));
#12530=CARTESIAN_POINT('Origin',(-13.112465101899,14.8031072225088,-25.0483789742253));
#12531=CARTESIAN_POINT('',(-15.112465101899,14.8031072225088,-25.0483789742253));
#12532=CARTESIAN_POINT('',(-15.112465101899,14.8031072225088,-25.0483789742253));
#12533=CARTESIAN_POINT('Origin',(-13.112465101899,14.8031072225088,-25.0483789742253));
#12534=CARTESIAN_POINT('Origin',(-8.07921903294852,6.34965048929021,-41.0483789742253));
#12535=CARTESIAN_POINT('Origin',(-0.499999999999999,25.4362251590507,-25.0483789742253));
#12536=CARTESIAN_POINT('',(-0.499999999999999,-6.43177298256785,-25.0483789742253));
#12537=CARTESIAN_POINT('',(-0.499999999999999,25.4362251590507,-25.0483789742253));
#12538=CARTESIAN_POINT('',(-20.5,-6.43177298256785,-25.0483789742253));
#12539=CARTESIAN_POINT('',(-0.499999999999999,-6.43177298256785,-25.0483789742253));
#12540=CARTESIAN_POINT('',(-20.5,25.4362251590507,-25.0483789742253));
#12541=CARTESIAN_POINT('',(-20.5,17.4692256236461,-25.0483789742253));
#12542=CARTESIAN_POINT('',(-0.499999999999999,25.4362251590507,-25.0483789742253));
#12543=CARTESIAN_POINT('',(-14.7402854682776,22.2688065021356,-25.0483789742253));
#12544=CARTESIAN_POINT('',(0.620142734138823,22.2688065021356,-25.0483789742253));
#12545=CARTESIAN_POINT('',(-15.7402854682776,21.2688065021356,-25.0483789742253));
#12546=CARTESIAN_POINT('Origin',(-14.7402854682776,21.2688065021356,-25.0483789742253));
#12547=CARTESIAN_POINT('',(-15.7402854682776,17.8031073387245,-25.0483789742253));
#12548=CARTESIAN_POINT('',(-15.7402854682776,23.3525158305932,-25.0483789742253));
#12549=CARTESIAN_POINT('Origin',(-14.7402854682776,17.8031073387245,-25.0483789742253));
#12550=CARTESIAN_POINT('',(-15.112465101899,11.6662094575612,-25.0483789742253));
#12551=CARTESIAN_POINT('Origin',(-15.112465101899,6.43177298256785,-32.9865355928432));
#12552=CARTESIAN_POINT('',(-15.112465101899,10.4317729825678,-32.9865355928432));
#12553=CARTESIAN_POINT('Origin',(-15.112465101899,6.43177298256785,-32.9865355928432));
#12554=CARTESIAN_POINT('',(-15.112465101899,10.4317729825678,-32.9865355928432));
#12555=CARTESIAN_POINT('Origin',(-15.112465101899,-2.10380624392837,-25.0483789742253));
#12556=CARTESIAN_POINT('Origin',(1.74028546827764,22.2688065021356,-25.0483789742253));
#12557=CARTESIAN_POINT('',(-14.7402854682776,22.2688065021356,-20.2341199955735));
#12558=CARTESIAN_POINT('',(-0.499999999999999,22.2688065021356,-20.2341199955735));
#12559=CARTESIAN_POINT('',(-14.7402854682776,22.2688065021356,-25.0483789742253));
#12560=CARTESIAN_POINT('Origin',(-15.7402854682776,21.2688065021356,-25.0483789742253));
#12561=CARTESIAN_POINT('',(-15.7402854682776,21.2688065021356,-23.0483789742253));
#12562=CARTESIAN_POINT('',(-15.7402854682776,21.2688065021356,-25.0483789742253));
#12563=CARTESIAN_POINT('',(-15.7402854682776,17.8031073387245,-23.0483789742253));
#12564=CARTESIAN_POINT('',(-15.7402854682776,23.3525158305932,-23.0483789742253));
#12565=CARTESIAN_POINT('',(-15.7402854682776,17.8031073387245,-25.0483789742253));
#12566=CARTESIAN_POINT('Origin',(-14.7402854682776,21.2688065021356,-25.0483789742253));
#12567=CARTESIAN_POINT('',(-15.694331048449,21.5684680294553,-23.0483789742253));
#12568=CARTESIAN_POINT('Ctrl Pts',(-15.694331048449,21.5684680294553,-23.0483789742253));
#12569=CARTESIAN_POINT('Ctrl Pts',(-15.7067045333496,21.5290740215346,-22.8358435371785));
#12570=CARTESIAN_POINT('Ctrl Pts',(-15.7107993314416,21.5098518119976,-22.6191838880156));
#12571=CARTESIAN_POINT('Ctrl Pts',(-15.7107993314416,21.5098518119976,-22.0465473119767));
#12572=CARTESIAN_POINT('Ctrl Pts',(-15.7017461665905,21.5718168405896,-21.6587360262855));
#12573=CARTESIAN_POINT('Ctrl Pts',(-15.6217540845814,21.7453252007984,-21.1350970538315));
#12574=CARTESIAN_POINT('Ctrl Pts',(-15.5832369350269,21.8154399994892,-20.9705071584932));
#12575=CARTESIAN_POINT('Ctrl Pts',(-15.4627032474283,21.9670099916972,-20.6729862218086));
#12576=CARTESIAN_POINT('Ctrl Pts',(-15.3825634860813,22.048920053459,-20.5395299428976));
#12577=CARTESIAN_POINT('Ctrl Pts',(-15.1938793645158,22.1631936845831,-20.3730368907704));
#12578=CARTESIAN_POINT('Ctrl Pts',(-15.1132023218396,22.201380934103,-20.3213948743704));
#12579=CARTESIAN_POINT('Ctrl Pts',(-14.9336495994831,22.2543889579894,-20.2519607649698));
#12580=CARTESIAN_POINT('Ctrl Pts',(-14.8346739441802,22.2688065021356,-20.2341199955735));
#12581=CARTESIAN_POINT('Ctrl Pts',(-14.7402854682776,22.2688065021356,-20.2341199955735));
#12582=CARTESIAN_POINT('Origin',(-14.7402854682776,21.2688065021356,-23.0483789742253));
#12583=CARTESIAN_POINT('Origin',(-14.7402854682776,17.8031073387245,-25.0483789742253));
#12584=CARTESIAN_POINT('Origin',(-14.7402854682776,17.8031073387245,-23.0483789742253));
#12585=CARTESIAN_POINT('Origin',(-0.499999999999999,9.50222608824143,11.9189153104842));
#12586=CARTESIAN_POINT('',(-0.499999999999999,-2.56401585297239,-23.0483789742253));
#12587=CARTESIAN_POINT('',(-0.499999999999999,17.4692256236461,-23.0483789742253));
#12588=CARTESIAN_POINT('',(-0.499999999999999,-6.43177298256785,-18.9365770263474));
#12589=CARTESIAN_POINT('Origin',(-0.499999999999999,-6.00539963551477,-22.4105093470644));
#12590=CARTESIAN_POINT('',(-0.499999999999999,-6.43177298256785,26.0826265387027));
#12591=CARTESIAN_POINT('',(-0.499999999999999,-6.43177298256785,-5.56473183187052));
#12592=CARTESIAN_POINT('',(-0.499999999999999,-6.43177298256785,33.0141314097479));
#12593=CARTESIAN_POINT('Origin',(-0.499999999999999,-5.94334688204796,29.5483789742253));
#12594=CARTESIAN_POINT('',(-0.499999999999999,-6.43177298256785,46.8862095951938));
#12595=CARTESIAN_POINT('',(-0.499999999999999,-6.43177298256785,-5.56473183187052));
#12596=CARTESIAN_POINT('',(-0.499999999999999,-5.56822701743215,46.8862095951938));
#12597=CARTESIAN_POINT('',(-0.499999999999999,1.53522655283679,46.8862095951938));
#12598=CARTESIAN_POINT('',(-0.499999999999999,-5.56822701743215,48.8862095951938));
#12599=CARTESIAN_POINT('',(-0.499999999999999,-5.56822701743215,30.402562452839));
#12600=CARTESIAN_POINT('',(-0.499999999999999,-6.43177298256785,48.8862095951938));
#12601=CARTESIAN_POINT('',(-0.499999999999999,-6.43177298256785,48.8862095951938));
#12602=CARTESIAN_POINT('',(-0.499999999999999,-8.43177298256785,46.8862095951938));
#12603=CARTESIAN_POINT('Origin',(-0.499999999999999,-6.43177298256785,46.8862095951938));
#12604=CARTESIAN_POINT('',(-0.499999999999999,-8.43177298256785,-23.0483789742253));
#12605=CARTESIAN_POINT('',(-0.499999999999999,-8.43177298256785,-23.0483789742253));
#12606=CARTESIAN_POINT('Origin',(-0.499999999999999,-6.43177298256785,-23.0483789742253));
#12607=CARTESIAN_POINT('',(-0.499999999999999,-7.44334688204796,29.5483789742253));
#12608=CARTESIAN_POINT('Origin',(-0.499999999999999,-5.94334688204796,29.5483789742253));
#12609=CARTESIAN_POINT('',(-0.499999999999999,-7.50539963551477,-22.4105093470644));
#12610=CARTESIAN_POINT('Origin',(-0.499999999999999,-6.00539963551477,-22.4105093470644));
#12611=CARTESIAN_POINT('Origin',(-16.5,-3.56822701743215,48.8862095951938));
#12612=CARTESIAN_POINT('',(-18.5,-3.56822701743215,46.8862095951938));
#12613=CARTESIAN_POINT('',(-16.5,-5.56822701743215,46.8862095951938));
#12614=CARTESIAN_POINT('Origin',(-16.5,-3.56822701743215,46.8862095951938));
#12615=CARTESIAN_POINT('',(-18.5,-3.56822701743215,48.8862095951938));
#12616=CARTESIAN_POINT('',(-18.5,-3.56822701743215,48.8862095951938));
#12617=CARTESIAN_POINT('',(-16.5,-5.56822701743215,48.8862095951938));
#12618=CARTESIAN_POINT('Origin',(-16.5,-3.56822701743215,48.8862095951938));
#12619=CARTESIAN_POINT('',(-16.5,-5.56822701743215,48.8862095951938));
#12620=CARTESIAN_POINT('Origin',(3.5,-5.56822701743215,48.8862095951938));
#12621=CARTESIAN_POINT('',(1.5,-5.56822701743215,46.8862095951938));
#12622=CARTESIAN_POINT('',(1.5,-5.56822701743215,48.8862095951938));
#12623=CARTESIAN_POINT('Origin',(-16.5,18.4317729825679,48.8862095951938));
#12624=CARTESIAN_POINT('',(-16.5,18.4317729825679,46.8862095951938));
#12625=CARTESIAN_POINT('',(-8.5,18.4317729825679,46.8862095951938));
#12626=CARTESIAN_POINT('',(-16.5,18.4317729825679,48.8862095951938));
#12627=CARTESIAN_POINT('',(-8.5,18.4317729825679,48.8862095951938));
#12628=CARTESIAN_POINT('',(-16.5,18.4317729825679,48.8862095951938));
#12629=CARTESIAN_POINT('Origin',(-16.5,16.4317729825679,48.8862095951938));
#12630=CARTESIAN_POINT('',(-18.5,16.4317729825679,46.8862095951938));
#12631=CARTESIAN_POINT('Origin',(-16.5,16.4317729825679,46.8862095951938));
#12632=CARTESIAN_POINT('',(-18.5,16.4317729825679,48.8862095951938));
#12633=CARTESIAN_POINT('Origin',(-16.5,16.4317729825679,48.8862095951938));
#12634=CARTESIAN_POINT('',(-18.5,16.4317729825679,48.8862095951938));
#12635=CARTESIAN_POINT('Origin',(-18.5,-3.56822701743215,48.8862095951938));
#12636=CARTESIAN_POINT('',(-18.5,-5.,46.8862095951938));
#12637=CARTESIAN_POINT('',(-18.5,-5.,48.8862095951938));
#12638=CARTESIAN_POINT('Origin',(-0.499999999999999,-6.43177298256785,48.8862095951938));
#12639=CARTESIAN_POINT('',(-20.5,19.2953189477036,48.8862095951938));
#12640=CARTESIAN_POINT('',(-0.499999999999999,19.2953189477036,48.8862095951938));
#12641=CARTESIAN_POINT('',(-20.5,-6.43177298256785,48.8862095951938));
#12642=CARTESIAN_POINT('',(-20.5,1.53522655283679,48.8862095951938));
#12643=CARTESIAN_POINT('',(-0.499999999999999,-6.43177298256785,48.8862095951938));
#12644=CARTESIAN_POINT('Origin',(-0.499999999999999,25.4362251590507,-23.0483789742253));
#12645=CARTESIAN_POINT('',(-19.5,21.5684680294553,-23.0483789742253));
#12646=CARTESIAN_POINT('',(-0.499999999999999,21.5684680294553,-23.0483789742253));
#12647=CARTESIAN_POINT('',(-19.5,-2.56401585297239,-23.0483789742253));
#12648=CARTESIAN_POINT('',(-19.5,17.4692256236461,-23.0483789742253));
#12649=CARTESIAN_POINT('',(-0.499999999999999,-2.56401585297239,-23.0483789742253));
#12650=CARTESIAN_POINT('Origin',(-19.5,9.50222608824143,11.9189153104842));
#12651=CARTESIAN_POINT('',(-19.5,25.4362251590507,-18.9365770263474));
#12652=CARTESIAN_POINT('Origin',(-19.5,25.0098518119976,-22.4105093470644));
#12653=CARTESIAN_POINT('',(-19.5,25.4362251590507,26.0826265387027));
#12654=CARTESIAN_POINT('',(-19.5,25.4362251590507,20.9642631075063));
#12655=CARTESIAN_POINT('',(-19.5,21.4945386978003,30.1184604429708));
#12656=CARTESIAN_POINT('Origin',(-19.5,24.9477990585308,29.5483789742253));
#12657=CARTESIAN_POINT('',(-19.5,19.2953189477036,33.0096109045284));
#12658=CARTESIAN_POINT('Origin',(-19.5,22.2953189477035,33.0096109045284));
#12659=CARTESIAN_POINT('',(-19.5,19.2953189477036,46.8862095951938));
#12660=CARTESIAN_POINT('',(-19.5,19.2953189477035,29.402562452839));
#12661=CARTESIAN_POINT('',(-19.5,-6.43177298256785,46.8862095951938));
#12662=CARTESIAN_POINT('',(-19.5,1.53522655283679,46.8862095951938));
#12663=CARTESIAN_POINT('',(-19.5,-6.43177298256785,33.0141314097479));
#12664=CARTESIAN_POINT('',(-19.5,-6.43177298256785,-5.56473183187052));
#12665=CARTESIAN_POINT('',(-19.5,-6.43177298256785,26.0826265387027));
#12666=CARTESIAN_POINT('Origin',(-19.5,-5.94334688204796,29.5483789742253));
#12667=CARTESIAN_POINT('',(-19.5,-6.43177298256785,-18.9365770263474));
#12668=CARTESIAN_POINT('',(-19.5,-6.43177298256785,-5.56473183187052));
#12669=CARTESIAN_POINT('Origin',(-19.5,-6.00539963551477,-22.4105093470644));
#12670=CARTESIAN_POINT('Origin',(-0.499999999999999,25.4362251590507,30.0096109045284));
#12671=CARTESIAN_POINT('',(-0.499999999999999,25.4362251590507,-18.9365770263474));
#12672=CARTESIAN_POINT('',(-0.499999999999999,25.4362251590507,26.0826265387027));
#12673=CARTESIAN_POINT('Origin',(-0.499999999999999,-6.43177298256785,-23.0483789742253));
#12674=CARTESIAN_POINT('',(-0.499999999999999,-6.43177298256785,33.0141314097479));
#12675=CARTESIAN_POINT('',(-0.499999999999999,-6.43177298256785,46.8862095951938));
#12676=CARTESIAN_POINT('Origin',(-0.499999999999999,-6.43177298256785,-23.0483789742253));
#12677=CARTESIAN_POINT('',(-0.499999999999999,-6.43177298256785,26.0826265387027));
#12678=CARTESIAN_POINT('',(-0.499999999999999,-6.43177298256785,-18.9365770263474));
#12679=CARTESIAN_POINT('Origin',(-0.499999999999999,22.2953189477035,33.0096109045284));
#12680=CARTESIAN_POINT('',(-0.499999999999999,21.4945386978003,30.1184604429708));
#12681=CARTESIAN_POINT('',(-0.499999999999999,19.2953189477036,33.0096109045284));
#12682=CARTESIAN_POINT('Origin',(-0.499999999999999,-6.43177298256785,46.8862095951938));
#12683=CARTESIAN_POINT('',(-0.499999999999999,19.2953189477036,46.8862095951938));
#12684=CARTESIAN_POINT('Origin',(-0.499999999999999,24.9477990585308,29.5483789742253));
#12685=CARTESIAN_POINT('Origin',(-0.499999999999999,-6.00539963551477,-22.4105093470644));
#12686=CARTESIAN_POINT('Origin',(-0.499999999999999,-5.94334688204796,29.5483789742253));
#12687=CARTESIAN_POINT('Origin',(-0.499999999999999,25.0098518119976,-22.4105093470644));
#12688=CARTESIAN_POINT('Origin',(-0.499999999999999,19.2953189477036,46.8862095951938));
#12689=CARTESIAN_POINT('Origin',(-0.499999999999999,24.9477990585308,29.5483789742253));
#12690=CARTESIAN_POINT('',(-18.5,23.4477990585308,29.5483789742253));
#12691=CARTESIAN_POINT('',(-0.499999999999999,23.4477990585308,29.5483789742253));
#12692=CARTESIAN_POINT('Origin',(-18.5,24.9477990585308,29.5483789742253));
#12693=CARTESIAN_POINT('Origin',(-18.5,24.9477990585308,29.5483789742253));
#12694=CARTESIAN_POINT('Origin',(-0.499999999999999,-6.00539963551477,-22.4105093470644));
#12695=CARTESIAN_POINT('',(-18.5,-7.50539963551477,-22.4105093470644));
#12696=CARTESIAN_POINT('',(-0.499999999999999,-7.50539963551477,-22.4105093470644));
#12697=CARTESIAN_POINT('Origin',(-18.5,-6.00539963551477,-22.4105093470644));
#12698=CARTESIAN_POINT('Origin',(-18.5,-6.00539963551477,-22.4105093470644));
#12699=CARTESIAN_POINT('Origin',(-0.499999999999999,-5.94334688204796,29.5483789742253));
#12700=CARTESIAN_POINT('',(-18.5,-7.44334688204796,29.5483789742253));
#12701=CARTESIAN_POINT('',(-0.499999999999999,-7.44334688204796,29.5483789742253));
#12702=CARTESIAN_POINT('Origin',(-18.5,-5.94334688204796,29.5483789742253));
#12703=CARTESIAN_POINT('Origin',(-18.5,-5.94334688204796,29.5483789742253));
#12704=CARTESIAN_POINT('Origin',(-0.499999999999999,25.0098518119976,-22.4105093470644));
#12705=CARTESIAN_POINT('',(-18.5,23.5098518119976,-22.4105093470644));
#12706=CARTESIAN_POINT('',(-0.499999999999999,23.5098518119976,-22.4105093470644));
#12707=CARTESIAN_POINT('Origin',(-18.5,25.0098518119976,-22.4105093470644));
#12708=CARTESIAN_POINT('Origin',(-18.5,25.0098518119976,-22.4105093470644));
#12709=CARTESIAN_POINT('Origin',(-20.5,20.2953189477035,29.402562452839));
#12710=CARTESIAN_POINT('',(-21.5,20.2953189477036,46.8862095951938));
#12711=CARTESIAN_POINT('',(-20.5,21.2953189477036,46.8862095951938));
#12712=CARTESIAN_POINT('Origin',(-20.5,20.2953189477036,46.8862095951938));
#12713=CARTESIAN_POINT('',(-20.5,21.2953189477036,33.0096109045284));
#12714=CARTESIAN_POINT('',(-20.5,21.2953189477035,29.402562452839));
#12715=CARTESIAN_POINT('',(-21.5,20.2953189477035,33.0096109045284));
#12716=CARTESIAN_POINT('Origin',(-20.5,20.2953189477035,33.0096109045284));
#12717=CARTESIAN_POINT('',(-21.5,20.2953189477035,29.402562452839));
#12718=CARTESIAN_POINT('Origin',(-20.5,22.2953189477035,33.0096109045284));
#12719=CARTESIAN_POINT('',(-20.5,22.2953189477036,32.0096109045284));
#12720=CARTESIAN_POINT('',(-21.5,22.2953189477036,31.0096109045284));
#12721=CARTESIAN_POINT('Origin',(-20.5,22.2953189477036,31.0096109045284));
#12722=CARTESIAN_POINT('Origin',(-21.5,22.2953189477035,33.0096109045284));
#12723=CARTESIAN_POINT('Origin',(-20.5,22.2953189477035,33.0096109045284));
#12724=CARTESIAN_POINT('Origin',(-20.5,15.8987725179725,31.0096109045284));
#12725=CARTESIAN_POINT('',(-20.5,25.4362251590507,32.0096109045284));
#12726=CARTESIAN_POINT('',(-21.5,25.4362251590507,31.0096109045284));
#12727=CARTESIAN_POINT('Origin',(-20.5,25.4362251590507,31.0096109045284));
#12728=CARTESIAN_POINT('',(-21.5,15.8987725179725,31.0096109045284));
#12729=CARTESIAN_POINT('',(-20.5,15.8987725179725,32.0096109045284));
#12730=CARTESIAN_POINT('Ctrl Pts',(-20.5,25.4362251590507,32.0096109045284));
#12731=CARTESIAN_POINT('Ctrl Pts',(-20.5,27.4362251590507,32.0096109045285));
#12732=CARTESIAN_POINT('Ctrl Pts',(-20.5,27.4362251590507,30.0096109045284));
#12733=CARTESIAN_POINT('Ctrl Pts',(-21.5,25.4362251590507,32.0096109045284));
#12734=CARTESIAN_POINT('Ctrl Pts',(-21.5,27.4362251590507,32.0096109045285));
#12735=CARTESIAN_POINT('Ctrl Pts',(-21.5,27.4362251590507,30.0096109045284));
#12736=CARTESIAN_POINT('Ctrl Pts',(-21.5,25.4362251590507,31.0096109045284));
#12737=CARTESIAN_POINT('Ctrl Pts',(-21.5,26.4362251590507,31.0096109045284));
#12738=CARTESIAN_POINT('Ctrl Pts',(-21.5,26.4362251590507,30.0096109045284));
#12739=CARTESIAN_POINT('',(-20.5,27.4362251590507,30.0096109045284));
#12740=CARTESIAN_POINT('',(-21.5,26.4362251590507,30.0096109045284));
#12741=CARTESIAN_POINT('Origin',(-20.5,26.4362251590507,30.0096109045284));
#12742=CARTESIAN_POINT('Origin',(-21.5,25.4362251590507,30.0096109045284));
#12743=CARTESIAN_POINT('Origin',(-20.5,25.4362251590507,30.0096109045284));
#12744=CARTESIAN_POINT('Origin',(-20.5,26.4362251590507,20.9642631075063));
#12745=CARTESIAN_POINT('',(-20.5,27.4362251590507,-23.0483789742253));
#12746=CARTESIAN_POINT('',(-21.5,26.4362251590507,-23.0483789742253));
#12747=CARTESIAN_POINT('Origin',(-20.5,26.4362251590507,-23.0483789742253));
#12748=CARTESIAN_POINT('',(-21.5,26.4362251590507,20.9642631075063));
#12749=CARTESIAN_POINT('',(-20.5,27.4362251590507,20.9642631075063));
#12750=CARTESIAN_POINT('Ctrl Pts',(-20.5,27.4362251590507,-23.0483789742253));
#12751=CARTESIAN_POINT('Ctrl Pts',(-20.5,27.4362251590507,-25.0483789742253));
#12752=CARTESIAN_POINT('Ctrl Pts',(-20.5,25.4362251590507,-25.0483789742253));
#12753=CARTESIAN_POINT('Ctrl Pts',(-21.5,27.4362251590507,-23.0483789742253));
#12754=CARTESIAN_POINT('Ctrl Pts',(-21.5,27.4362251590507,-25.0483789742253));
#12755=CARTESIAN_POINT('Ctrl Pts',(-21.5,25.4362251590507,-25.0483789742253));
#12756=CARTESIAN_POINT('Ctrl Pts',(-21.5,26.4362251590507,-23.0483789742253));
#12757=CARTESIAN_POINT('Ctrl Pts',(-21.5,26.4362251590507,-24.0483789742253));
#12758=CARTESIAN_POINT('Ctrl Pts',(-21.5,25.4362251590507,-24.0483789742253));
#12759=CARTESIAN_POINT('',(-21.5,25.4362251590507,-24.0483789742253));
#12760=CARTESIAN_POINT('Origin',(-20.5,25.4362251590507,-24.0483789742253));
#12761=CARTESIAN_POINT('Origin',(-21.5,25.4362251590507,-23.0483789742253));
#12762=CARTESIAN_POINT('Origin',(-20.5,25.4362251590507,-23.0483789742253));
#12763=CARTESIAN_POINT('Origin',(-20.5,17.4692256236461,-24.0483789742253));
#12764=CARTESIAN_POINT('',(-21.5,-6.43177298256785,-24.0483789742253));
#12765=CARTESIAN_POINT('Origin',(-20.5,-6.43177298256785,-24.0483789742253));
#12766=CARTESIAN_POINT('',(-21.5,17.4692256236461,-24.0483789742253));
#12767=CARTESIAN_POINT('Ctrl Pts',(-20.5,-6.43177298256785,-25.0483789742253));
#12768=CARTESIAN_POINT('Ctrl Pts',(-20.5,-8.43177298256785,-25.0483789742253));
#12769=CARTESIAN_POINT('Ctrl Pts',(-20.5,-8.43177298256785,-23.0483789742253));
#12770=CARTESIAN_POINT('Ctrl Pts',(-21.5,-6.43177298256785,-25.0483789742253));
#12771=CARTESIAN_POINT('Ctrl Pts',(-21.5,-8.43177298256785,-25.0483789742253));
#12772=CARTESIAN_POINT('Ctrl Pts',(-21.5,-8.43177298256785,-23.0483789742253));
#12773=CARTESIAN_POINT('Ctrl Pts',(-21.5,-6.43177298256785,-24.0483789742253));
#12774=CARTESIAN_POINT('Ctrl Pts',(-21.5,-7.43177298256785,-24.0483789742253));
#12775=CARTESIAN_POINT('Ctrl Pts',(-21.5,-7.43177298256785,-23.0483789742253));
#12776=CARTESIAN_POINT('',(-20.5,-8.43177298256785,-23.0483789742253));
#12777=CARTESIAN_POINT('',(-21.5,-7.43177298256785,-23.0483789742253));
#12778=CARTESIAN_POINT('Origin',(-20.5,-7.43177298256785,-23.0483789742253));
#12779=CARTESIAN_POINT('Origin',(-21.5,-6.43177298256785,-23.0483789742253));
#12780=CARTESIAN_POINT('Origin',(-20.5,-6.43177298256785,-23.0483789742253));
#12781=CARTESIAN_POINT('Origin',(-20.5,-7.43177298256785,-5.56473183187052));
#12782=CARTESIAN_POINT('',(-20.5,-8.43177298256785,46.8862095951938));
#12783=CARTESIAN_POINT('',(-21.5,-7.43177298256786,46.8862095951938));
#12784=CARTESIAN_POINT('Origin',(-20.5,-7.43177298256786,46.8862095951938));
#12785=CARTESIAN_POINT('',(-21.5,-7.43177298256785,-5.56473183187052));
#12786=CARTESIAN_POINT('',(-20.5,-8.43177298256785,-5.56473183187052));
#12787=CARTESIAN_POINT('Ctrl Pts',(-20.5,-8.43177298256785,46.8862095951938));
#12788=CARTESIAN_POINT('Ctrl Pts',(-20.5,-8.43177298256785,48.8862095951938));
#12789=CARTESIAN_POINT('Ctrl Pts',(-20.5,-6.43177298256785,48.8862095951938));
#12790=CARTESIAN_POINT('Ctrl Pts',(-21.5,-8.43177298256785,46.8862095951938));
#12791=CARTESIAN_POINT('Ctrl Pts',(-21.5,-8.43177298256785,48.8862095951938));
#12792=CARTESIAN_POINT('Ctrl Pts',(-21.5,-6.43177298256785,48.8862095951938));
#12793=CARTESIAN_POINT('Ctrl Pts',(-21.5,-7.43177298256786,46.8862095951938));
#12794=CARTESIAN_POINT('Ctrl Pts',(-21.5,-7.43177298256785,47.8862095951938));
#12795=CARTESIAN_POINT('Ctrl Pts',(-21.5,-6.43177298256785,47.8862095951938));
#12796=CARTESIAN_POINT('',(-21.5,-6.43177298256785,47.8862095951938));
#12797=CARTESIAN_POINT('Origin',(-20.5,-6.43177298256785,47.8862095951938));
#12798=CARTESIAN_POINT('Origin',(-21.5,-6.43177298256785,46.8862095951938));
#12799=CARTESIAN_POINT('Origin',(-20.5,-6.43177298256785,46.8862095951938));
#12800=CARTESIAN_POINT('Origin',(-20.5,1.53522655283679,47.8862095951938));
#12801=CARTESIAN_POINT('',(-21.5,19.2953189477036,47.8862095951938));
#12802=CARTESIAN_POINT('Origin',(-20.5,19.2953189477036,47.8862095951938));
#12803=CARTESIAN_POINT('',(-21.5,1.53522655283679,47.8862095951938));
#12804=CARTESIAN_POINT('Ctrl Pts',(-20.5,19.2953189477036,48.8862095951938));
#12805=CARTESIAN_POINT('Ctrl Pts',(-20.5,21.2953189477036,48.8862095951938));
#12806=CARTESIAN_POINT('Ctrl Pts',(-20.5,21.2953189477036,46.8862095951938));
#12807=CARTESIAN_POINT('Ctrl Pts',(-21.5,19.2953189477036,48.8862095951938));
#12808=CARTESIAN_POINT('Ctrl Pts',(-21.5,21.2953189477036,48.8862095951938));
#12809=CARTESIAN_POINT('Ctrl Pts',(-21.5,21.2953189477036,46.8862095951938));
#12810=CARTESIAN_POINT('Ctrl Pts',(-21.5,19.2953189477036,47.8862095951938));
#12811=CARTESIAN_POINT('Ctrl Pts',(-21.5,20.2953189477036,47.8862095951938));
#12812=CARTESIAN_POINT('Ctrl Pts',(-21.5,20.2953189477036,46.8862095951938));
#12813=CARTESIAN_POINT('Origin',(-21.5,19.2953189477036,46.8862095951938));
#12814=CARTESIAN_POINT('Origin',(-20.5,19.2953189477036,46.8862095951938));
#12815=CARTESIAN_POINT('Origin',(-0.499999999999999,25.4362251590507,-23.0483789742253));
#12816=CARTESIAN_POINT('',(-0.499999999999999,27.4362251590507,-23.0483789742253));
#12817=CARTESIAN_POINT('Origin',(-0.499999999999999,27.4362251590507,30.0096109045284));
#12818=CARTESIAN_POINT('',(-0.499999999999999,27.4362251590507,30.0096109045284));
#12819=CARTESIAN_POINT('Origin',(-0.499999999999999,25.4362251590507,30.0096109045284));
#12820=CARTESIAN_POINT('',(-0.499999999999999,25.4362251590507,32.0096109045284));
#12821=CARTESIAN_POINT('Origin',(-0.499999999999999,22.2953189477036,32.0096109045284));
#12822=CARTESIAN_POINT('',(-0.499999999999999,22.2953189477036,32.0096109045284));
#12823=CARTESIAN_POINT('Origin',(-0.499999999999999,22.2953189477035,33.0096109045284));
#12824=CARTESIAN_POINT('',(-0.499999999999999,21.2953189477036,33.0096109045284));
#12825=CARTESIAN_POINT('Origin',(-0.499999999999999,21.2953189477036,46.8862095951938));
#12826=CARTESIAN_POINT('',(-0.499999999999999,21.2953189477036,46.8862095951938));
#12827=CARTESIAN_POINT('Origin',(-21.5,9.50222608824143,11.9189153104842));
#12828=CARTESIAN_POINT('Origin',(-0.499999999999999,19.2953189477036,46.8862095951938));
#12829=CARTESIAN_POINT('Origin',(-0.499999999999999,-6.43177298256785,46.8862095951938));
#12830=CARTESIAN_POINT('',(-0.499999999999999,-8.43177298256785,46.8862095951938));
#12831=CARTESIAN_POINT('Origin',(-0.499999999999999,-8.43177298256785,-23.0483789742253));
#12832=CARTESIAN_POINT('',(-0.499999999999999,-8.43177298256785,-23.0483789742253));
#12833=CARTESIAN_POINT('Origin',(-0.499999999999999,-6.43177298256785,-23.0483789742253));
#17017=UNCERTAINTY_MEASURE_WITH_UNIT(LENGTH_MEASURE(0.01),#17043,
'DISTANCE_ACCURACY_VALUE',
'Maximum model space distance between geometric entities at asserted c
onnectivities');
#17028=UNCERTAINTY_MEASURE_WITH_UNIT(LENGTH_MEASURE(0.01),#17043,
'DISTANCE_ACCURACY_VALUE',
'Maximum model space distance between geometric entities at asserted c
onnectivities');
#17031=(
GEOMETRIC_REPRESENTATION_CONTEXT(3)
GLOBAL_UNCERTAINTY_ASSIGNED_CONTEXT((#17017))
GLOBAL_UNIT_ASSIGNED_CONTEXT((#17043,#17045,#17046))
REPRESENTATION_CONTEXT('','3D')
);
#17042=(
GEOMETRIC_REPRESENTATION_CONTEXT(3)
GLOBAL_UNCERTAINTY_ASSIGNED_CONTEXT((#17028))
GLOBAL_UNIT_ASSIGNED_CONTEXT((#17043,#17045,#17046))
REPRESENTATION_CONTEXT('','3D')
);
#17043=(
LENGTH_UNIT()
NAMED_UNIT(*)
SI_UNIT(.MILLI.,.METRE.)
);
#17045=(
NAMED_UNIT(*)
PLANE_ANGLE_UNIT()
SI_UNIT($,.RADIAN.)
);
#17046=(
NAMED_UNIT(*)
SI_UNIT($,.STERADIAN.)
SOLID_ANGLE_UNIT()
);
#17049=SHAPE_DEFINITION_REPRESENTATION(#17062,#17087);
#17062=PRODUCT_DEFINITION_SHAPE('',$,#17101);
#17087=SHAPE_REPRESENTATION('',(#8462),#17031);
#17098=PRODUCT_DEFINITION_CONTEXT('part definition',#17139,'design');
#17101=PRODUCT_DEFINITION('CLAMSHELL_BOT','CLAMSHELL_BOT',#17114,#17098);
#17114=PRODUCT_DEFINITION_FORMATION('',$,#17143);
#17139=APPLICATION_CONTEXT(
'Core Data for Automotive Mechanical Design Process');
#17140=PRODUCT_CONTEXT('part definition',#17139,'mechanical');
#17143=PRODUCT('CLAMSHELL_BOT','CLAMSHELL_BOT',$,(#17140));
#17154=PRESENTATION_STYLE_ASSIGNMENT((#17155));
#17155=SURFACE_STYLE_USAGE(.BOTH.,#17156);
#17156=SURFACE_SIDE_STYLE('',(#17157));
#17157=SURFACE_STYLE_FILL_AREA(#17158);
#17158=FILL_AREA_STYLE('Steel - Satin',(#17159));
#17159=FILL_AREA_STYLE_COLOUR('Steel - Satin',#17160);
#17160=COLOUR_RGB('Steel - Satin', 0.09019608, 0.27058824, 0.51372549);
ENDSEC;
END-ISO-10303-21;
